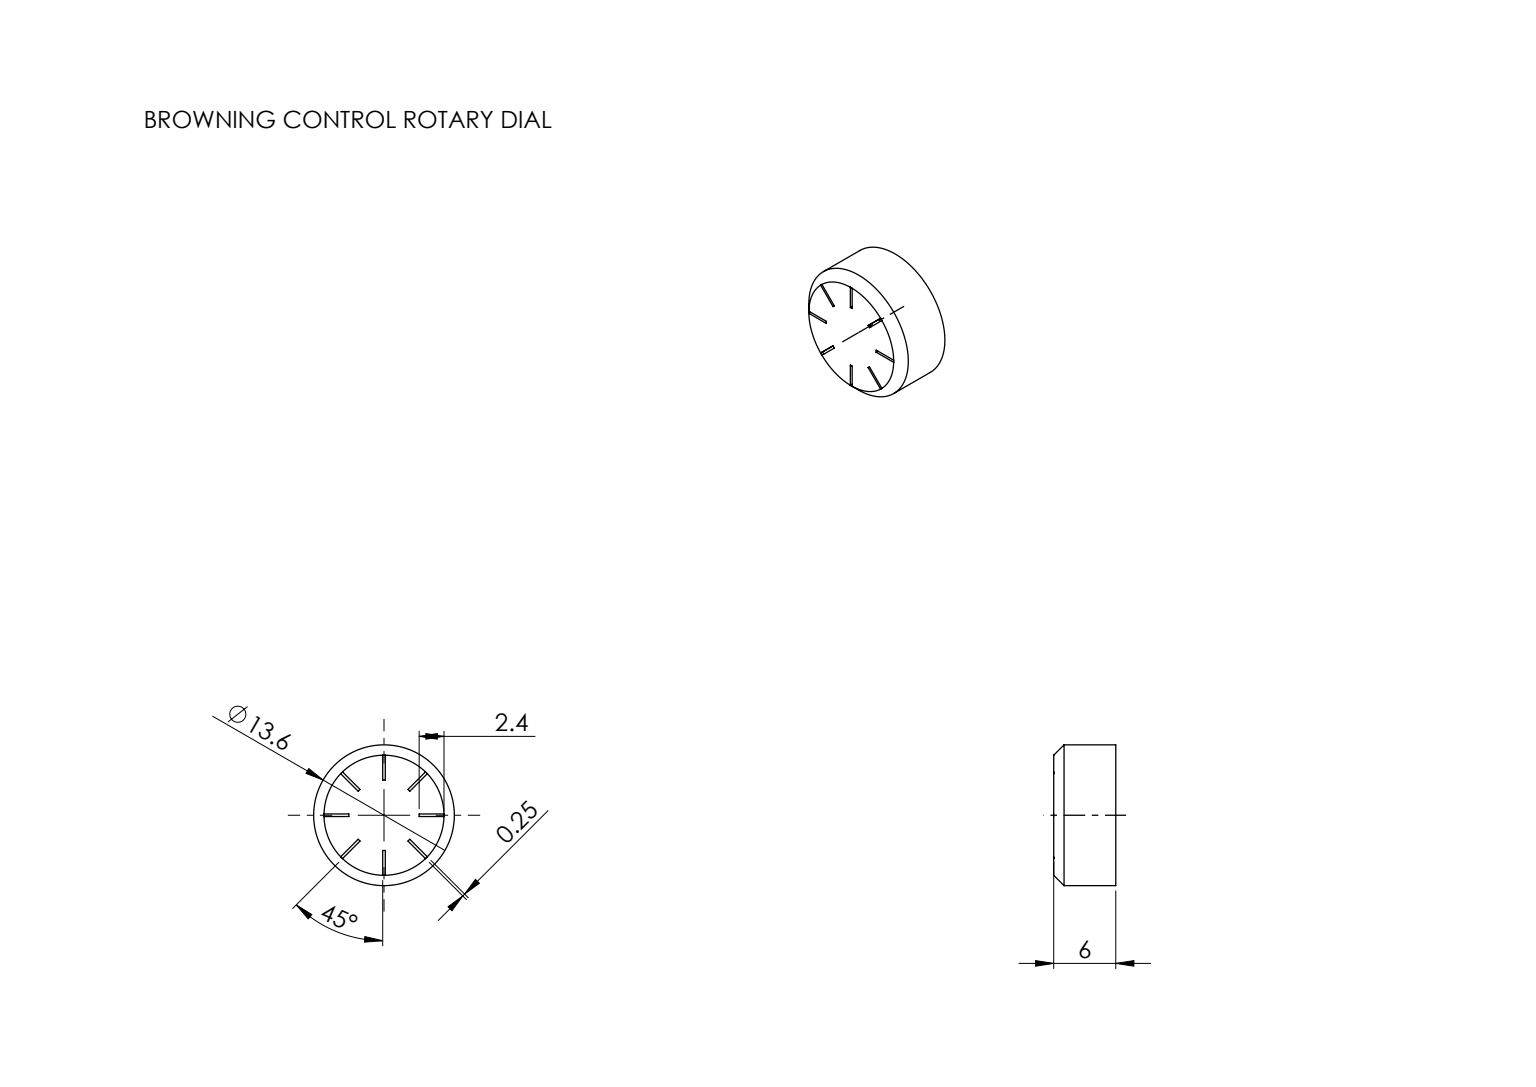
ISO-10303-21;
HEADER;
FILE_DESCRIPTION (('STEP AP214'),
    '1' );
FILE_NAME ('Browning Control Rotary Dial.step',
    '2026-10-08T14:41:38',
    ( '' ),
    ( '' ),
    'SwSTEP 2.0',
    'SolidWorks 2026',
    '' );
FILE_SCHEMA (( 'AUTOMOTIVE_DESIGN' ));
ENDSEC;

DATA;
#38=AXIS2_PLACEMENT_3D ( 'NONE', #15476, #386, #16855 ) ;
#44=EDGE_CURVE ( 'NONE', #885, #4327, #14471, .T. ) ;
#48=B_SPLINE_CURVE_WITH_KNOTS ( 'NONE', 3,
 ( #13537, #4634, #4733, #16687 ),
 .UNSPECIFIED., .F., .F.,
 ( 4, 4 ),
 ( 0.000000000000000000, 1.000000000000000000 ),
 .UNSPECIFIED. ) ;
#78=ADVANCED_FACE ( 'NONE', ( #3019 ), #8997, .T. ) ;
#88=CLOSED_SHELL ( 'NONE', ( #433, #16433, #12643, #3854, #16960, #8083, #12476, #2887, #13363, #11571, #11070, #10821, #5435, #14081, #18479, #16340, #3288, #10464, #13954, #1717, #18414, #1458, #6350, #11815, #16187, #14084, #2136, #6137, #1464, #12159, #2663, #1129, #18269, #562, #5420, #78, #10177, #12810, #725, #8545, #7974, #4556, #12238, #18488, #11655, #2010 ) ) ;
#89=VERTEX_POINT ( 'NONE', #13508 ) ;
#93=CARTESIAN_POINT ( 'NONE',  ( 4.072081901468762588, 26.82127119883315558, 59.66337542264481186 ) ) ;
#97=ORIENTED_EDGE ( 'NONE', *, *, #1658, .T. ) ;
#106=VERTEX_POINT ( 'NONE', #9669 ) ;
#125=CARTESIAN_POINT ( 'NONE',  ( 4.101219330881969327, 32.64264068711926825, 53.84264068711931372 ) ) ;
#154=PLANE ( 'NONE',  #4763 ) ;
#166=DIRECTION ( 'NONE',  ( 0.000000000000000000, -0.7071067811865495711, 0.7071067811865454633 ) ) ;
#181=ORIENTED_EDGE ( 'NONE', *, *, #18284, .T. ) ;
#182=ORIENTED_EDGE ( 'NONE', *, *, #1003, .F. ) ;
#191=CARTESIAN_POINT ( 'NONE',  ( 4.012354697599916697, 26.78000129688588871, 59.70432772728319293 ) ) ;
#212=ORIENTED_EDGE ( 'NONE', *, *, #12916, .T. ) ;
#217=EDGE_CURVE ( 'NONE', #3132, #14286, #15567, .T. ) ;
#224=ORIENTED_EDGE ( 'NONE', *, *, #676, .F. ) ;
#231=PLANE ( 'NONE',  #3745 ) ;
#237=DIRECTION ( 'NONE',  ( -0.7071067811865512365, -0.4999999999999988898, 0.4999999999999959477 ) ) ;
#239=DIRECTION ( 'NONE',  ( 0.7071067811865513475, 0.4999999999999988898, -0.4999999999999959477 ) ) ;
#256=DIRECTION ( 'NONE',  ( 0.000000000000000000, 0.7071067811865490160, -0.7071067811865461294 ) ) ;
#267=LINE ( 'NONE', #6253, #11429 ) ;
#275=DIRECTION ( 'NONE',  ( 0.000000000000000000, 0.7071067811865456854, 0.7071067811865494601 ) ) ;
#286=ORIENTED_EDGE ( 'NONE', *, *, #17624, .F. ) ;
#290=EDGE_LOOP ( 'NONE', ( #1568, #17362, #14195, #8849 ) ) ;
#305=ORIENTED_EDGE ( 'NONE', *, *, #2220, .F. ) ;
#314=EDGE_CURVE ( 'NONE', #106, #11781, #3884, .T. ) ;
#327=EDGE_CURVE ( 'NONE', #16495, #6094, #13076, .T. ) ;
#336=CARTESIAN_POINT ( 'NONE',  ( -1.084502282093227498E-14, 29.65425233947093986, 56.83102903476761725 ) ) ;
#357=CARTESIAN_POINT ( 'NONE',  ( -4.189607678530257395, 32.40336399182267257, 53.72836399182263278 ) ) ;
#386=DIRECTION ( 'NONE',  ( 0.000000000000000000, 0.7071067811865456854, 0.7071067811865494601 ) ) ;
#389=EDGE_LOOP ( 'NONE', ( #6259, #18026, #496, #1957 ) ) ;
#398=AXIS2_PLACEMENT_3D ( 'NONE', #14982, #7531, #3118 ) ;
#415=ORIENTED_EDGE ( 'NONE', *, *, #7089, .T. ) ;
#433=ADVANCED_FACE ( 'NONE', ( #10043 ), #844, .T. ) ;
#468=ORIENTED_EDGE ( 'NONE', *, *, #1195, .F. ) ;
#475=DIRECTION ( 'NONE',  ( -0.7071067811865511255, -0.4999999999999987788, 0.4999999999999958922 ) ) ;
#496=ORIENTED_EDGE ( 'NONE', *, *, #14059, .F. ) ;
#515=AXIS2_PLACEMENT_3D ( 'NONE', #7618, #13582, #166 ) ;
#521=CARTESIAN_POINT ( 'NONE',  ( 0.1249999999999895917, 33.84386001800125143, 52.64142135623733765 ) ) ;
#527=DIRECTION ( 'NONE',  ( -1.942890293094023946E-16, 0.7071067811865453523, 0.7071067811865496822 ) ) ;
#533=CARTESIAN_POINT ( 'NONE',  ( 4.101219330881941794, 26.84264068711924267, 59.64264068711931088 ) ) ;
#545=EDGE_CURVE ( 'NONE', #16762, #576, #17802, .T. ) ;
#562=ADVANCED_FACE ( 'NONE', ( #8873 ), #154, .T. ) ;
#563=ORIENTED_EDGE ( 'NONE', *, *, #6960, .T. ) ;
#576=VERTEX_POINT ( 'NONE', #13377 ) ;
#582=DIRECTION ( 'NONE',  ( 2.220446049250312834E-16, 0.7071067811865455743, 0.7071067811865493491 ) ) ;
#591=CARTESIAN_POINT ( 'NONE',  ( 5.799999999999985612, 29.65425233947092920, 56.47747564417436195 ) ) ;
#598=CARTESIAN_POINT ( 'NONE',  ( 5.799999999999985612, 29.65425233947092920, 56.47747564417436195 ) ) ;
#602=ORIENTED_EDGE ( 'NONE', *, *, #4334, .F. ) ;
#609=AXIS2_PLACEMENT_3D ( 'NONE', #15894, #14234, #2648 ) ;
#666=CARTESIAN_POINT ( 'NONE',  ( 5.799999999999985612, 29.65425233947092920, 56.47747564417436195 ) ) ;
#671=COLOUR_RGB ( '', 0.72549020, 0.75294118, 0.79215686) ;
#676=EDGE_CURVE ( 'NONE', #9708, #9275, #13573, .T. ) ;
#693=CARTESIAN_POINT ( 'NONE',  ( -1.040834085586084257E-14, 29.03553390593270578, 56.03553390593273775 ) ) ;
#704=CARTESIAN_POINT ( 'NONE',  ( -4.012354697599906928, 32.70432772728319293, 53.78000129688592068 ) ) ;
#705=CARTESIAN_POINT ( 'NONE',  ( -0.1250000000000104083, 31.97002704785689531, 54.16170093578840294 ) ) ;
#706=EDGE_CURVE ( 'NONE', #9890, #18408, #2462, .T. ) ;
#716=CARTESIAN_POINT ( 'NONE',  ( -2.492551403682565780, 31.20336399182265552, 54.92836399182263563 ) ) ;
#725=ADVANCED_FACE ( 'NONE', ( #16824 ), #4868, .T. ) ;
#742=DIRECTION ( 'NONE',  ( -1.000000000000000000, 2.720046410331633524E-15, -2.220446049250313081E-15 ) ) ;
#750=ORIENTED_EDGE ( 'NONE', *, *, #15854, .T. ) ;
#779=ORIENTED_EDGE ( 'NONE', *, *, #9790, .T. ) ;
#789=FACE_OUTER_BOUND ( 'NONE', #10775, .T. ) ;
#807=FACE_OUTER_BOUND ( 'NONE', #12482, .T. ) ;
#816=ORIENTED_EDGE ( 'NONE', *, *, #9598, .T. ) ;
#835=SURFACE_STYLE_FILL_AREA ( #11035 ) ;
#842=ORIENTED_EDGE ( 'NONE', *, *, #15989, .T. ) ;
#843=FACE_OUTER_BOUND ( 'NONE', #12229, .T. ) ;
#844=CYLINDRICAL_SURFACE ( 'NONE', #14759, 6.799999999999997158 ) ;
#852=LINE ( 'NONE', #17325, #17405 ) ;
#861=EDGE_CURVE ( 'NONE', #12841, #2217, #5438, .T. ) ;
#872=DIRECTION ( 'NONE',  ( 0.5773502691896360561, 0.8164965809277188180, 0.000000000000000000 ) ) ;
#881=ORIENTED_EDGE ( 'NONE', *, *, #9499, .T. ) ;
#885=VERTEX_POINT ( 'NONE', #10021 ) ;
#889=CARTESIAN_POINT ( 'NONE',  ( 0.1249999999999895917, 27.16170093578836031, 58.97002704785691662 ) ) ;
#895=VERTEX_POINT ( 'NONE', #3865 ) ;
#903=DIRECTION ( 'NONE',  ( 1.000000000000000000, -7.410738689372937262E-15, 7.410738689372897819E-15 ) ) ;
#914=DIRECTION ( 'NONE',  ( 1.000000000000000000, -2.665111688417744333E-15, 2.272588573746785565E-15 ) ) ;
#989=CARTESIAN_POINT ( 'NONE',  ( -5.799326430397251819, 29.65377616443625541, 56.83055285973284754 ) ) ;
#990=ORIENTED_EDGE ( 'NONE', *, *, #7649, .F. ) ;
#1003=EDGE_CURVE ( 'NONE', #16765, #16368, #9344, .T. ) ;
#1051=ORIENTED_EDGE ( 'NONE', *, *, #5788, .F. ) ;
#1061=DIRECTION ( 'NONE',  ( -0.000000000000000000, 0.7071067811865493491, -0.7071067811865456854 ) ) ;
#1068=CARTESIAN_POINT ( 'NONE',  ( -9.575581032440643243E-15, 20.69167388793145079, 57.30832611206850657 ) ) ;
#1072=ORIENTED_EDGE ( 'NONE', *, *, #15999, .T. ) ;
#1092=EDGE_CURVE ( 'NONE', #2343, #576, #12483, .T. ) ;
#1097=ORIENTED_EDGE ( 'NONE', *, *, #3003, .F. ) ;
#1128=AXIS2_PLACEMENT_3D ( 'NONE', #9817, #18860, #10100 ) ;
#1129=ADVANCED_FACE ( 'NONE', ( #7187 ), #13161, .F. ) ;
#1140=CARTESIAN_POINT ( 'NONE',  ( 4.189607678530260948, 26.72836399182260791, 59.40336399182267257 ) ) ;
#1157=CARTESIAN_POINT ( 'NONE',  ( -4.160453206537193083, 26.88344170207934525, 59.60057016663802187 ) ) ;
#1163=CARTESIAN_POINT ( 'NONE',  ( -5.800000000000006928, 29.47747564417435484, 56.65425233947093631 ) ) ;
#1169=ORIENTED_EDGE ( 'NONE', *, *, #14932, .T. ) ;
#1170=ORIENTED_EDGE ( 'NONE', *, *, #17994, .F. ) ;
#1175=DIRECTION ( 'NONE',  ( 0.7071067811865388020, -0.5000000000000074385, 0.5000000000000046629 ) ) ;
#1176=ORIENTED_EDGE ( 'NONE', *, *, #1238, .T. ) ;
#1185=SHAPE_DEFINITION_REPRESENTATION ( #6159, #2502 ) ;
#1189=LINE ( 'NONE', #8840, #18689 ) ;
#1191=ORIENTED_EDGE ( 'NONE', *, *, #676, .T. ) ;
#1195=EDGE_CURVE ( 'NONE', #4388, #12056, #11985, .T. ) ;
#1201=DIRECTION ( 'NONE',  ( -2.775557561562890858E-16, 0.7071067811865456854, 0.7071067811865493491 ) ) ;
#1221=DIRECTION ( 'NONE',  ( -0.5773502691896282846, -0.8164965809277242581, 0.000000000000000000 ) ) ;
#1231=CARTESIAN_POINT ( 'NONE',  ( 0.1249999999999895917, 25.46464466094064250, 60.66708332270462734 ) ) ;
#1232=DIRECTION ( 'NONE',  ( 0.7071067811865414665, -0.5000000000000058842, 0.5000000000000028866 ) ) ;
#1235=LINE ( 'NONE', #1140, #3481 ) ;
#1238=EDGE_CURVE ( 'NONE', #3008, #10469, #14216, .T. ) ;
#1256=EDGE_LOOP ( 'NONE', ( #16470, #14104, #2812, #8914 ) ) ;
#1263=DIRECTION ( 'NONE',  ( 0.000000000000000000, -0.7071067811865452413, -0.7071067811865497932 ) ) ;
#1268=CARTESIAN_POINT ( 'NONE',  ( -0.1250000000000104083, 27.33847763108499507, 59.14680374315354783 ) ) ;
#1292=CARTESIAN_POINT ( 'NONE',  ( -2.492551403682614186, 28.10514068711927749, 58.38014068711927251 ) ) ;
#1297=CARTESIAN_POINT ( 'NONE',  ( -2.315774708385926139, 31.50514068711928672, 54.98014068711927393 ) ) ;
#1325=VECTOR ( 'NONE', #4373, 1000.000000000000114 ) ;
#1339=B_SPLINE_CURVE_WITH_KNOTS ( 'NONE', 3,
 ( #8067, #10986, #6398, #704 ),
 .UNSPECIFIED., .F., .F.,
 ( 4, 4 ),
 ( 0.000000000000000000, 1.000000000000000000 ),
 .UNSPECIFIED. ) ;
#1340=DIRECTION ( 'NONE',  ( 0.000000000000000000, -0.7071067811865457964, -0.7071067811865492381 ) ) ;
#1349=ORIENTED_EDGE ( 'NONE', *, *, #2635, .F. ) ;
#1357=ORIENTED_EDGE ( 'NONE', *, *, #4764, .F. ) ;
#1360=EDGE_CURVE ( 'NONE', #16495, #18191, #17257, .T. ) ;
#1375=EDGE_LOOP ( 'NONE', ( #3971, #16864, #9192, #16577, #12901 ) ) ;
#1378=CARTESIAN_POINT ( 'NONE',  ( -4.012354697599992193, 26.78000129688593134, 59.70432772728315740 ) ) ;
#1388=CARTESIAN_POINT ( 'NONE',  ( -4.189607678530257395, 32.40336399182267257, 53.72836399182263278 ) ) ;
#1432=DIRECTION ( 'NONE',  ( 1.000000000000000000, 0.000000000000000000, -0.000000000000000000 ) ) ;
#1447=VERTEX_POINT ( 'NONE', #12922 ) ;
#1458=ADVANCED_FACE ( 'NONE', ( #15877 ), #16253, .F. ) ;
#1463=CARTESIAN_POINT ( 'NONE',  ( 4.101219330881969327, 32.64264068711926825, 53.84264068711931372 ) ) ;
#1464=ADVANCED_FACE ( 'NONE', ( #18916 ), #11445, .T. ) ;
#1486=ORIENTED_EDGE ( 'NONE', *, *, #7089, .F. ) ;
#1491=CARTESIAN_POINT ( 'NONE',  ( -0.1250000000000104083, 25.46464466094064250, 60.66708332270462734 ) ) ;
#1539=LINE ( 'NONE', #7513, #3636 ) ;
#1555=LINE ( 'NONE', #17724, #16314 ) ;
#1559=CARTESIAN_POINT ( 'NONE',  ( 2.315774708385922587, 27.80336399182260720, 58.32836399182267684 ) ) ;
#1562=CARTESIAN_POINT ( 'NONE',  ( 4.042620306204053549, 26.80012125920691446, 59.68389060951044200 ) ) ;
#1564=EDGE_CURVE ( 'NONE', #16934, #16046, #11536, .T. ) ;
#1568=ORIENTED_EDGE ( 'NONE', *, *, #12470, .F. ) ;
#1607=VERTEX_POINT ( 'NONE', #1463 ) ;
#1640=AXIS2_PLACEMENT_3D ( 'NONE', #2314, #2693, #1221 ) ;
#1658=EDGE_CURVE ( 'NONE', #6570, #18891, #1755, .T. ) ;
#1664=FACE_OUTER_BOUND ( 'NONE', #7252, .T. ) ;
#1669=ORIENTED_EDGE ( 'NONE', *, *, #17624, .T. ) ;
#1688=CARTESIAN_POINT ( 'NONE',  ( -0.1250000000000104083, 25.46464466094064250, 60.66708332270462734 ) ) ;
#1692=EDGE_LOOP ( 'NONE', ( #8443, #17446, #17916, #6022 ) ) ;
#1694=CARTESIAN_POINT ( 'NONE',  ( 0.000000000000000000, 43.06586399182256741, 43.06586399182279479 ) ) ;
#1700=LINE ( 'NONE', #15233, #14879 ) ;
#1702=EDGE_CURVE ( 'NONE', #16934, #9890, #16362, .T. ) ;
#1708=FACE_OUTER_BOUND ( 'NONE', #5051, .T. ) ;
#1714=EDGE_CURVE ( 'NONE', #13315, #14325, #16755, .T. ) ;
#1717=ADVANCED_FACE ( 'NONE', ( #1664 ), #14985, .T. ) ;
#1724=DIRECTION ( 'NONE',  ( 0.7071067811865513475, 0.4999999999999988898, -0.4999999999999959477 ) ) ;
#1755=LINE ( 'NONE', #19303, #8738 ) ;
#1789=VERTEX_POINT ( 'NONE', #4898 ) ;
#1791=AXIS2_PLACEMENT_3D ( 'NONE', #13713, #4815, #7646 ) ;
#1801=LINE ( 'NONE', #3561, #9692 ) ;
#1809=VERTEX_POINT ( 'NONE', #18426 ) ;
#1810=B_SPLINE_CURVE_WITH_KNOTS ( 'NONE', 3,
 ( #6841, #15227, #8048, #2057 ),
 .UNSPECIFIED., .F., .F.,
 ( 4, 4 ),
 ( 0.000000000000000000, 1.000000000000000000 ),
 .UNSPECIFIED. ) ;
#1812=EDGE_CURVE ( 'NONE', #17726, #12801, #3518, .T. ) ;
#1823=DIRECTION ( 'NONE',  ( -0.5773502691896228445, 0.8164965809277280329, 0.000000000000000000 ) ) ;
#1830=DIRECTION ( 'NONE',  ( -0.7071067811865437980, 0.5000000000000039968, -0.5000000000000013323 ) ) ;
#1901=DIRECTION ( 'NONE',  ( -0.7071067811865537900, -0.4999999999999972800, 0.4999999999999940603 ) ) ;
#1957=ORIENTED_EDGE ( 'NONE', *, *, #3607, .F. ) ;
#1965=AXIS2_PLACEMENT_3D ( 'NONE', #17931, #275, #5869 ) ;
#1973=FACE_OUTER_BOUND ( 'NONE', #5364, .T. ) ;
#2010=ADVANCED_FACE ( 'NONE', ( #14469 ), #14659, .T. ) ;
#2035=ORIENTED_EDGE ( 'NONE', *, *, #2635, .T. ) ;
#2043=CARTESIAN_POINT ( 'NONE',  ( -2.315774708385978098, 27.80336399182263563, 58.32836399182264131 ) ) ;
#2051=VECTOR ( 'NONE', #14820, 1000.000000000000000 ) ;
#2057=CARTESIAN_POINT ( 'NONE',  ( 5.799326430397229615, 29.65377616443619857, 56.83055285973290438 ) ) ;
#2067=LINE ( 'NONE', #7958, #15703 ) ;
#2078=DIRECTION ( 'NONE',  ( -7.602811950582247805E-15, 0.000000000000000000, 1.000000000000000000 ) ) ;
#2080=VERTEX_POINT ( 'NONE', #12985 ) ;
#2093=ORIENTED_EDGE ( 'NONE', *, *, #11143, .F. ) ;
#2094=DIRECTION ( 'NONE',  ( 8.659560562354847809E-17, -1.000000000000000000, -1.221245327087672194E-14 ) ) ;
#2097=DIRECTION ( 'NONE',  ( 0.000000000000000000, 0.7071067811865456854, 0.7071067811865494601 ) ) ;
#2119=CARTESIAN_POINT ( 'NONE',  ( -3.400000000000017675, 29.47747564417433352, 56.65425233947095052 ) ) ;
#2136=ADVANCED_FACE ( 'NONE', ( #8678 ), #2411, .F. ) ;
#2188=CARTESIAN_POINT ( 'NONE',  ( 4.012830983233651061, 32.52836399182262994, 53.60336399182268252 ) ) ;
#2191=CARTESIAN_POINT ( 'NONE',  ( -13.49999999999974065, 39.11180553784110003, 47.01992244580424085 ) ) ;
#2195=CIRCLE ( 'NONE', #4064, 6.799999999999999822 ) ;
#2201=FACE_OUTER_BOUND ( 'NONE', #18242, .T. ) ;
#2217=VERTEX_POINT ( 'NONE', #6047 ) ;
#2220=EDGE_CURVE ( 'NONE', #10469, #11653, #13483, .T. ) ;
#2236=DIRECTION ( 'NONE',  ( -2.220446049250312588E-16, 0.7071067811865453523, 0.7071067811865496822 ) ) ;
#2243=ORIENTED_EDGE ( 'NONE', *, *, #4334, .T. ) ;
#2261=CARTESIAN_POINT ( 'NONE',  ( -4.189131392896543460, 32.57932772728320003, 53.90500129688591358 ) ) ;
#2279=ORIENTED_EDGE ( 'NONE', *, *, #9499, .F. ) ;
#2281=VERTEX_POINT ( 'NONE', #13274 ) ;
#2288=CARTESIAN_POINT ( 'NONE',  ( 2.492551403682577771, 31.20336399182262710, 54.92836399182266405 ) ) ;
#2295=CARTESIAN_POINT ( 'NONE',  ( -0.1250000000000104083, 27.33847763108499507, 59.14680374315354783 ) ) ;
#2304=CARTESIAN_POINT ( 'NONE',  ( 5.800448907431066559, 29.80092238452519382, 56.68308948419219462 ) ) ;
#2314=CARTESIAN_POINT ( 'NONE',  ( 4.012830983233651061, 32.52836399182262994, 53.60336399182268252 ) ) ;
#2343=VERTEX_POINT ( 'NONE', #8203 ) ;
#2355=PRODUCT_DEFINITION_FORMATION_WITH_SPECIFIED_SOURCE ( 'ANY', '', #17717, .NOT_KNOWN. ) ;
#2371=DIRECTION ( 'NONE',  ( 0.5773502691896202910, -0.8164965809277299202, 0.000000000000000000 ) ) ;
#2373=CARTESIAN_POINT ( 'NONE',  ( -2.492551403682614186, 27.92836399182264273, 58.20336399182264131 ) ) ;
#2382=EDGE_LOOP ( 'NONE', ( #2833, #842, #12674, #5103 ) ) ;
#2386=CARTESIAN_POINT ( 'NONE',  ( -3.400000000000017675, 29.65425233947097183, 56.47747564417432642 ) ) ;
#2399=LINE ( 'NONE', #17121, #17102 ) ;
#2400=ORIENTED_EDGE ( 'NONE', *, *, #2495, .T. ) ;
#2411=PLANE ( 'NONE',  #15954 ) ;
#2417=ORIENTED_EDGE ( 'NONE', *, *, #8519, .T. ) ;
#2432=EDGE_CURVE ( 'NONE', #4388, #16762, #11119, .T. ) ;
#2447=VECTOR ( 'NONE', #6633, 999.9999999999998863 ) ;
#2462=CIRCLE ( 'NONE', #15927, 5.800000000000007816 ) ;
#2485=CARTESIAN_POINT ( 'NONE',  ( -5.800448837981397432, 29.77177811653248796, 56.71286850494549014 ) ) ;
#2495=EDGE_CURVE ( 'NONE', #2080, #15466, #3013, .T. ) ;
#2502=SHAPE_REPRESENTATION ( 'Browning Control Rotary Dial', ( #1791 ), #2636 ) ;
#2503=DIRECTION ( 'NONE',  ( 0.000000000000000000, 0.7071067811865456854, 0.7071067811865494601 ) ) ;
#2521=ORIENTED_EDGE ( 'NONE', *, *, #16911, .F. ) ;
#2544=ORIENTED_EDGE ( 'NONE', *, *, #706, .F. ) ;
#2549=EDGE_CURVE ( 'NONE', #5878, #3990, #9749, .T. ) ;
#2556=ORIENTED_EDGE ( 'NONE', *, *, #4085, .T. ) ;
#2562=VECTOR ( 'NONE', #7706, 1000.000000000000000 ) ;
#2578=CARTESIAN_POINT ( 'NONE',  ( -2.315774708385926139, 31.32836399182264842, 54.80336399182263563 ) ) ;
#2607=ORIENTED_EDGE ( 'NONE', *, *, #14511, .T. ) ;
#2635=EDGE_CURVE ( 'NONE', #9275, #12801, #2195, .T. ) ;
#2636=( GEOMETRIC_REPRESENTATION_CONTEXT ( 3 ) GLOBAL_UNCERTAINTY_ASSIGNED_CONTEXT ( ( #16291 ) ) GLOBAL_UNIT_ASSIGNED_CONTEXT ( ( #11213, #5357, #8294 ) ) REPRESENTATION_CONTEXT ( 'NONE', 'WORKASPACE' ) );
#2648=DIRECTION ( 'NONE',  ( -2.665111688417744333E-15, -1.000000000000000000, 0.000000000000000000 ) ) ;
#2654=AXIS2_PLACEMENT_3D ( 'NONE', #5320, #4141, #13134 ) ;
#2657=EDGE_CURVE ( 'NONE', #895, #7943, #12290, .T. ) ;
#2662=ORIENTED_EDGE ( 'NONE', *, *, #15902, .T. ) ;
#2663=ADVANCED_FACE ( 'NONE', ( #6513 ), #18184, .T. ) ;
#2672=CARTESIAN_POINT ( 'NONE',  ( 4.160453206537142457, 32.60057016663802187, 53.88344170207938788 ) ) ;
#2690=VERTEX_POINT ( 'NONE', #7653 ) ;
#2693=DIRECTION ( 'NONE',  ( -0.7071067811865463515, 0.5000000000000024425, -0.4999999999999993339 ) ) ;
#2696=CONICAL_SURFACE ( 'NONE', #13654, 5.800000000000005151, 0.7853981633974385090 ) ;
#2701=DIRECTION ( 'NONE',  ( -0.000000000000000000, -0.7071067811865456854, -0.7071067811865494601 ) ) ;
#2711=ORIENTED_EDGE ( 'NONE', *, *, #9387, .F. ) ;
#2730=CARTESIAN_POINT ( 'NONE',  ( -0.1250000000000104083, 27.16170093578836031, 58.97002704785691662 ) ) ;
#2767=DIRECTION ( 'NONE',  ( 0.7071067811865512365, 0.4999999999999988898, -0.4999999999999959477 ) ) ;
#2769=DIRECTION ( 'NONE',  ( 0.000000000000000000, -0.7071067811865454633, -0.7071067811865496822 ) ) ;
#2772=PLANE ( 'NONE',  #13601 ) ;
#2774=CARTESIAN_POINT ( 'NONE',  ( 0.1249999999999895917, 25.46464466094064250, 60.66708332270462734 ) ) ;
#2781=CARTESIAN_POINT ( 'NONE',  ( -5.799326430397249155, 29.83055285973289372, 56.65377616443620212 ) ) ;
#2811=CARTESIAN_POINT ( 'NONE',  ( -9.971658890789427512E-15, 29.83102903476757817, 56.65425233947097894 ) ) ;
#2812=ORIENTED_EDGE ( 'NONE', *, *, #3312, .T. ) ;
#2819=ORIENTED_EDGE ( 'NONE', *, *, #8356, .F. ) ;
#2822=ORIENTED_EDGE ( 'NONE', *, *, #14511, .F. ) ;
#2823=ORIENTED_EDGE ( 'NONE', *, *, #14262, .F. ) ;
#2825=DIRECTION ( 'NONE',  ( 0.000000000000000000, -0.7071067811865497932, 0.7071067811865452413 ) ) ;
#2826=DIRECTION ( 'NONE',  ( 0.000000000000000000, -0.7071067811865454633, -0.7071067811865496822 ) ) ;
#2833=ORIENTED_EDGE ( 'NONE', *, *, #14108, .F. ) ;
#2883=DIRECTION ( 'NONE',  ( -2.775557561562890858E-16, 0.7071067811865454633, 0.7071067811865496822 ) ) ;
#2887=ADVANCED_FACE ( 'NONE', ( #10384 ), #11750, .T. ) ;
#2895=CARTESIAN_POINT ( 'NONE',  ( 0.1249999999999895917, 33.84290755733280065, 52.64142146683631296 ) ) ;
#2928=EDGE_CURVE ( 'NONE', #12056, #2690, #12635, .T. ) ;
#2929=CARTESIAN_POINT ( 'NONE',  ( 0.08838834764830766355, 29.80514068711926257, 56.68014068711929809 ) ) ;
#2930=CARTESIAN_POINT ( 'NONE',  ( -1.040834085586084257E-14, 33.84386001800124433, 51.22720779386423118 ) ) ;
#2950=PLANE ( 'NONE',  #16446 ) ;
#3003=EDGE_CURVE ( 'NONE', #17432, #18408, #4914, .T. ) ;
#3008=VERTEX_POINT ( 'NONE', #18544 ) ;
#3013=B_SPLINE_CURVE_WITH_KNOTS ( 'NONE', 3,
 ( #11207, #2485, #17481, #8287 ),
 .UNSPECIFIED., .F., .F.,
 ( 4, 4 ),
 ( 0.000000000000000000, 1.000000000000000000 ),
 .UNSPECIFIED. ) ;
#3016=ORIENTED_EDGE ( 'NONE', *, *, #9343, .F. ) ;
#3019=FACE_OUTER_BOUND ( 'NONE', #17852, .T. ) ;
#3063=CARTESIAN_POINT ( 'NONE',  ( 0.04165538583019261221, 25.64078660347668759, 60.84386001800125854 ) ) ;
#3086=CARTESIAN_POINT ( 'NONE',  ( -2.315774708385926139, 31.50514068711928672, 54.98014068711927393 ) ) ;
#3091=CARTESIAN_POINT ( 'NONE',  ( 0.1249999999999895917, 32.14680374315353362, 54.33847763108504125 ) ) ;
#3118=DIRECTION ( 'NONE',  ( -1.000000000000000000, 0.000000000000000000, 0.000000000000000000 ) ) ;
#3129=ORIENTED_EDGE ( 'NONE', *, *, #15264, .F. ) ;
#3131=CARTESIAN_POINT ( 'NONE',  ( -0.1250000000000104083, 33.66708332270461312, 52.46464466094069934 ) ) ;
#3132=VERTEX_POINT ( 'NONE', #18721 ) ;
#3160=STYLED_ITEM ( 'NONE', ( #4954 ), #10129 ) ;
#3165=CARTESIAN_POINT ( 'NONE',  ( 4.072081901468789233, 32.66337542264476923, 53.82127119883322308 ) ) ;
#3177=VECTOR ( 'NONE', #18325, 1000.000000000000114 ) ;
#3212=ORIENTED_EDGE ( 'NONE', *, *, #1238, .F. ) ;
#3220=ORIENTED_EDGE ( 'NONE', *, *, #15244, .T. ) ;
#3265=CARTESIAN_POINT ( 'NONE',  ( 2.315774708385941683, 31.32836399182263065, 54.80336399182266405 ) ) ;
#3270=LINE ( 'NONE', #521, #14377 ) ;
#3277=CARTESIAN_POINT ( 'NONE',  ( -13.50000000000003908, 20.01992244580436164, 66.11180553784085134 ) ) ;
#3280=( LENGTH_UNIT ( ) NAMED_UNIT ( * ) SI_UNIT ( .MILLI., .METRE. ) );
#3288=ADVANCED_FACE ( 'NONE', ( #18518 ), #8557, .F. ) ;
#3309=ORIENTED_EDGE ( 'NONE', *, *, #6175, .T. ) ;
#3312=EDGE_CURVE ( 'NONE', #13315, #11055, #8650, .T. ) ;
#3343=ORIENTED_EDGE ( 'NONE', *, *, #327, .T. ) ;
#3370=DIRECTION ( 'NONE',  ( -1.047444401652940007E-14, -0.7071067811865495711, 0.7071067811865454633 ) ) ;
#3422=EDGE_LOOP ( 'NONE', ( #2521, #2243, #13517, #11831 ) ) ;
#3427=ORIENTED_EDGE ( 'NONE', *, *, #16911, .T. ) ;
#3444=VECTOR ( 'NONE', #1201, 1000.000000000000114 ) ;
#3448=FACE_OUTER_BOUND ( 'NONE', #7421, .T. ) ;
#3459=AXIS2_PLACEMENT_3D ( 'NONE', #693, #6677, #16627 ) ;
#3462=ORIENTED_EDGE ( 'NONE', *, *, #12015, .F. ) ;
#3481=VECTOR ( 'NONE', #17234, 1000.000000000000000 ) ;
#3514=VECTOR ( 'NONE', #582, 1000.000000000000114 ) ;
#3517=FACE_OUTER_BOUND ( 'NONE', #7642, .T. ) ;
#3518=LINE ( 'NONE', #12706, #18159 ) ;
#3558=EDGE_LOOP ( 'NONE', ( #10549, #14712, #6356, #14505, #17843, #2544, #4769, #3309, #10055, #12014, #9614, #182, #6932, #5407, #8428 ) ) ;
#3561=CARTESIAN_POINT ( 'NONE',  ( -0.1250000000000104083, 27.16170093578836031, 58.97002704785691662 ) ) ;
#3564=CARTESIAN_POINT ( 'NONE',  ( -1.040834085586084257E-14, 25.49999999999998934, 52.50000000000000000 ) ) ;
#3607=EDGE_CURVE ( 'NONE', #19340, #17432, #18467, .T. ) ;
#3631=DIRECTION ( 'NONE',  ( 0.000000000000000000, 0.7071067811865490160, -0.7071067811865461294 ) ) ;
#3635=CARTESIAN_POINT ( 'NONE',  ( 3.399999999999996803, 29.47747564417430155, 56.65425233947098604 ) ) ;
#3636=VECTOR ( 'NONE', #12113, 1000.000000000000227 ) ;
#3655=ORIENTED_EDGE ( 'NONE', *, *, #5788, .T. ) ;
#3699=DIRECTION ( 'NONE',  ( -0.000000000000000000, -0.7071067811865456854, -0.7071067811865493491 ) ) ;
#3708=ORIENTED_EDGE ( 'NONE', *, *, #13973, .F. ) ;
#3714=PLANE ( 'NONE',  #9451 ) ;
#3745=AXIS2_PLACEMENT_3D ( 'NONE', #4252, #17774, #2769 ) ;
#3760=AXIS2_PLACEMENT_3D ( 'NONE', #16578, #16482, #10485 ) ;
#3765=VECTOR ( 'NONE', #15296, 1000.000000000000114 ) ;
#3786=ORIENTED_EDGE ( 'NONE', *, *, #6175, .F. ) ;
#3798=DIRECTION ( 'NONE',  ( 2.775557561562890858E-16, 0.7071067811865454633, 0.7071067811865496822 ) ) ;
#3825=DIRECTION ( 'NONE',  ( 3.491481338843133355E-15, 0.7071067811865495711, -0.7071067811865454633 ) ) ;
#3839=DIRECTION ( 'NONE',  ( 0.000000000000000000, -0.7071067811865495711, 0.7071067811865454633 ) ) ;
#3844=ORIENTED_EDGE ( 'NONE', *, *, #13213, .T. ) ;
#3854=ADVANCED_FACE ( 'NONE', ( #13423 ), #5995, .T. ) ;
#3855=DIRECTION ( 'NONE',  ( -0.5773502691896255090, 0.8164965809277261455, 0.000000000000000000 ) ) ;
#3865=CARTESIAN_POINT ( 'NONE',  ( 4.189607678530260948, 26.72836399182260791, 59.40336399182267257 ) ) ;
#3884=LINE ( 'NONE', #14467, #9743 ) ;
#3913=CARTESIAN_POINT ( 'NONE',  ( 4.012830983233625304, 26.60336399182260791, 59.52836399182266547 ) ) ;
#3914=DIRECTION ( 'NONE',  ( 0.5773502691896335026, 0.8164965809277204833, 0.000000000000000000 ) ) ;
#3964=AXIS2_PLACEMENT_3D ( 'NONE', #15505, #6775, #2078 ) ;
#3971=ORIENTED_EDGE ( 'NONE', *, *, #16201, .F. ) ;
#3980=ORIENTED_EDGE ( 'NONE', *, *, #11178, .T. ) ;
#3990=VERTEX_POINT ( 'NONE', #9505 ) ;
#4007=CARTESIAN_POINT ( 'NONE',  ( 0.1249999999999895917, 32.14680374315353362, 54.33847763108504125 ) ) ;
#4027=LINE ( 'NONE', #12754, #17835 ) ;
#4057=APPLICATION_CONTEXT ( 'automotive_design' ) ;
#4061=LINE ( 'NONE', #9751, #5852 ) ;
#4064=AXIS2_PLACEMENT_3D ( 'NONE', #3564, #2097, #7787 ) ;
#4065=ORIENTED_EDGE ( 'NONE', *, *, #17882, .T. ) ;
#4085=EDGE_CURVE ( 'NONE', #5200, #8744, #13461, .T. ) ;
#4088=ORIENTED_EDGE ( 'NONE', *, *, #17527, .F. ) ;
#4106=CARTESIAN_POINT ( 'NONE',  ( -4.130991513055715103, 32.62172003681460808, 53.86292658466337713 ) ) ;
#4127=ORIENTED_EDGE ( 'NONE', *, *, #15999, .F. ) ;
#4141=DIRECTION ( 'NONE',  ( -0.7071067811865562325, -0.4999999999999955036, 0.4999999999999924505 ) ) ;
#4150=ORIENTED_EDGE ( 'NONE', *, *, #7742, .F. ) ;
#4157=CARTESIAN_POINT ( 'NONE',  ( -4.189607678530257395, 32.40336399182267257, 53.72836399182263278 ) ) ;
#4194=ORIENTED_EDGE ( 'NONE', *, *, #13010, .F. ) ;
#4234=DIRECTION ( 'NONE',  ( 0.5773502691896311712, 0.8164965809277222597, 0.000000000000000000 ) ) ;
#4252=CARTESIAN_POINT ( 'NONE',  ( -5.800000000000006928, 29.65425233947099315, 56.47747564417430510 ) ) ;
#4301=CARTESIAN_POINT ( 'NONE',  ( -4.189131392896629613, 26.90500129688593134, 59.57932772728315030 ) ) ;
#4311=LINE ( 'NONE', #10467, #8937 ) ;
#4320=CARTESIAN_POINT ( 'NONE',  ( -0.08838834764833139457, 29.68014068711926257, 56.80514068711929809 ) ) ;
#4322=VERTEX_POINT ( 'NONE', #7236 ) ;
#4327=VERTEX_POINT ( 'NONE', #8895 ) ;
#4329=LINE ( 'NONE', #1292, #2051 ) ;
#4334=EDGE_CURVE ( 'NONE', #16046, #5763, #1555, .T. ) ;
#4353=EDGE_CURVE ( 'NONE', #17254, #2217, #12488, .T. ) ;
#4357=DIRECTION ( 'NONE',  ( 1.000000000000000000, 0.000000000000000000, -0.000000000000000000 ) ) ;
#4361=VECTOR ( 'NONE', #17532, 1000.000000000000000 ) ;
#4363=CARTESIAN_POINT ( 'NONE',  ( 4.101219330881941794, 26.84264068711924267, 59.64264068711931088 ) ) ;
#4365=ORIENTED_EDGE ( 'NONE', *, *, #2928, .T. ) ;
#4370=AXIS2_PLACEMENT_3D ( 'NONE', #14648, #17691, #10124 ) ;
#4373=DIRECTION ( 'NONE',  ( -0.7071067811865486830, -0.5000000000000005551, 0.4999999999999978351 ) ) ;
#4384=CARTESIAN_POINT ( 'NONE',  ( 5.799326430397229615, 29.65377616443619857, 56.83055285973290438 ) ) ;
#4388=VERTEX_POINT ( 'NONE', #11045 ) ;
#4390=CONICAL_SURFACE ( 'NONE', #16923, 5.800000000000005151, 0.7853981633974385090 ) ;
#4400=EDGE_LOOP ( 'NONE', ( #18506, #15112, #16402, #3016, #13450 ) ) ;
#4402=CARTESIAN_POINT ( 'NONE',  ( -4.130991513055792375, 26.86292658466339489, 59.62172003681457255 ) ) ;
#4406=DIRECTION ( 'NONE',  ( 2.220446049250313081E-16, 0.7071067811865452413, 0.7071067811865497932 ) ) ;
#4431=ORIENTED_EDGE ( 'NONE', *, *, #15127, .F. ) ;
#4437=DIRECTION ( 'NONE',  ( 1.000000000000000000, -7.410738689372937262E-15, 7.410738689372897819E-15 ) ) ;
#4439=LINE ( 'NONE', #1688, #10202 ) ;
#4460=DIRECTION ( 'NONE',  ( 0.000000000000000000, -0.7071067811865493491, 0.7071067811865457964 ) ) ;
#4486=EDGE_CURVE ( 'NONE', #895, #11055, #10752, .T. ) ;
#4525=DIRECTION ( 'NONE',  ( -0.000000000000000000, -0.7071067811865456854, -0.7071067811865494601 ) ) ;
#4530=DIRECTION ( 'NONE',  ( 1.047444401652940007E-14, 0.7071067811865495711, -0.7071067811865454633 ) ) ;
#4538=DIRECTION ( 'NONE',  ( -0.7071067811865463515, 0.5000000000000023315, -0.4999999999999994449 ) ) ;
#4556=ADVANCED_FACE ( 'NONE', ( #843 ), #12793, .F. ) ;
#4562=VECTOR ( 'NONE', #4633, 1000.000000000000114 ) ;
#4571=EDGE_CURVE ( 'NONE', #5689, #3132, #5949, .T. ) ;
#4575=DIRECTION ( 'NONE',  ( -0.000000000000000000, -0.7071067811865456854, -0.7071067811865493491 ) ) ;
#4618=B_SPLINE_CURVE_WITH_KNOTS ( 'NONE', 3,
 ( #11544, #11357, #6776, #15790 ),
 .UNSPECIFIED., .F., .F.,
 ( 4, 4 ),
 ( 0.000000000000000000, 1.000000000000000000 ),
 .UNSPECIFIED. ) ;
#4633=DIRECTION ( 'NONE',  ( -2.775557561562890858E-16, 0.7071067811865456854, 0.7071067811865493491 ) ) ;
#4634=CARTESIAN_POINT ( 'NONE',  ( -0.04166183285594760033, 33.84354264162095660, 52.64110397985704282 ) ) ;
#4639=DIRECTION ( 'NONE',  ( -0.000000000000000000, 0.7071067811865497932, -0.7071067811865452413 ) ) ;
#4666=LINE ( 'NONE', #10623, #1325 ) ;
#4717=ORIENTED_EDGE ( 'NONE', *, *, #1092, .T. ) ;
#4721=VECTOR ( 'NONE', #13894, 1000.000000000000000 ) ;
#4732=DIRECTION ( 'NONE',  ( -2.775557561562883462E-16, 0.7071067811865454633, 0.7071067811865495711 ) ) ;
#4733=CARTESIAN_POINT ( 'NONE',  ( -0.08332366571188480620, 33.84322526524066177, 52.64078660347674798 ) ) ;
#4737=VECTOR ( 'NONE', #17814, 1000.000000000000000 ) ;
#4738=CARTESIAN_POINT ( 'NONE',  ( -4.042620306204127267, 26.80012125920696064, 59.68389060951041358 ) ) ;
#4763=AXIS2_PLACEMENT_3D ( 'NONE', #7503, #1432, #7407 ) ;
#4764=EDGE_CURVE ( 'NONE', #4322, #12056, #7186, .T. ) ;
#4769=ORIENTED_EDGE ( 'NONE', *, *, #10982, .T. ) ;
#4791=EDGE_LOOP ( 'NONE', ( #3708, #3844, #17141, #5446, #1051 ) ) ;
#4805=ORIENTED_EDGE ( 'NONE', *, *, #13073, .T. ) ;
#4807=DIRECTION ( 'NONE',  ( 0.7071067811865414665, -0.5000000000000057732, 0.5000000000000028866 ) ) ;
#4815=DIRECTION ( 'NONE',  ( 0.000000000000000000, 0.000000000000000000, 1.000000000000000000 ) ) ;
#4827=DIRECTION ( 'NONE',  ( -0.000000000000000000, 0.7071067811865497932, -0.7071067811865452413 ) ) ;
#4847=CARTESIAN_POINT ( 'NONE',  ( -0.1250000000000104083, 27.16170093578836031, 58.97002704785691662 ) ) ;
#4851=AXIS2_PLACEMENT_3D ( 'NONE', #6420, #12582, #18576 ) ;
#4855=SURFACE_STYLE_USAGE ( .BOTH. , #12294 ) ;
#4868=PLANE ( 'NONE',  #15624 ) ;
#4891=ORIENTED_EDGE ( 'NONE', *, *, #1564, .F. ) ;
#4898=CARTESIAN_POINT ( 'NONE',  ( -2.492551403682614186, 28.10514068711927749, 58.38014068711927251 ) ) ;
#4907=EDGE_LOOP ( 'NONE', ( #2823, #14575, #18369, #4127, #15491 ) ) ;
#4914=LINE ( 'NONE', #9404, #15959 ) ;
#4925=DIRECTION ( 'NONE',  ( -0.000000000000000000, 0.7071067811865493491, -0.7071067811865456854 ) ) ;
#4953=LINE ( 'NONE', #15436, #15475 ) ;
#4954=PRESENTATION_STYLE_ASSIGNMENT (( #4855 ) ) ;
#4974=AXIS2_PLACEMENT_3D ( 'NONE', #16134, #11418, #8305 ) ;
#5015=DIRECTION ( 'NONE',  ( 0.000000000000000000, -0.7071067811865457964, -0.7071067811865492381 ) ) ;
#5023=DIRECTION ( 'NONE',  ( 1.110223024625156540E-16, 0.7071067811865455743, 0.7071067811865494601 ) ) ;
#5031=ORIENTED_EDGE ( 'NONE', *, *, #11769, .T. ) ;
#5039=ORIENTED_EDGE ( 'NONE', *, *, #9036, .T. ) ;
#5051=EDGE_LOOP ( 'NONE', ( #881, #11264, #6472, #779 ) ) ;
#5052=EDGE_CURVE ( 'NONE', #17270, #9938, #13728, .T. ) ;
#5061=EDGE_CURVE ( 'NONE', #6083, #9185, #6487, .T. ) ;
#5092=CARTESIAN_POINT ( 'NONE',  ( 4.012830983233651061, 32.52836399182262994, 53.60336399182268252 ) ) ;
#5103=ORIENTED_EDGE ( 'NONE', *, *, #5061, .F. ) ;
#5105=EDGE_LOOP ( 'NONE', ( #5985, #18335, #3220, #12115 ) ) ;
#5145=UNCERTAINTY_MEASURE_WITH_UNIT (LENGTH_MEASURE( 1.000000000000000082E-05 ), #3280, 'distance_accuracy_value', 'NONE');
#5181=EDGE_CURVE ( 'NONE', #7943, #13315, #14396, .T. ) ;
#5197=CARTESIAN_POINT ( 'NONE',  ( 2.492551403682558675, 27.92836399182260720, 58.20336399182267684 ) ) ;
#5199=DIRECTION ( 'NONE',  ( -0.000000000000000000, 0.7071067811865456854, 0.7071067811865493491 ) ) ;
#5200=VERTEX_POINT ( 'NONE', #2261 ) ;
#5206=FACE_OUTER_BOUND ( 'NONE', #4400, .T. ) ;
#5229=CARTESIAN_POINT ( 'NONE',  ( -0.1250000000000104083, 33.66708332270461312, 52.46464466094069934 ) ) ;
#5268=CARTESIAN_POINT ( 'NONE',  ( -1.040834085586084257E-14, 29.74264068711926257, 56.74264068711929809 ) ) ;
#5320=CARTESIAN_POINT ( 'NONE',  ( -4.012830983233618198, 32.52836399182267257, 53.60336399182263989 ) ) ;
#5327=CARTESIAN_POINT ( 'NONE',  ( -4.012830983233701687, 26.60336399182265055, 59.52836399182262994 ) ) ;
#5357=( NAMED_UNIT ( * ) PLANE_ANGLE_UNIT ( ) SI_UNIT ( $, .RADIAN. ) );
#5364=EDGE_LOOP ( 'NONE', ( #10754, #13809, #2711, #9469, #12213, #7654, #3655, #2400, #2819, #2556, #1072, #15373, #4150, #9302, #16672 ) ) ;
#5375=DIRECTION ( 'NONE',  ( -0.000000000000000000, 0.7071067811865452413, 0.7071067811865497932 ) ) ;
#5393=CARTESIAN_POINT ( 'NONE',  ( -4.189607678530337331, 26.72836399182265055, 59.40336399182262284 ) ) ;
#5394=ORIENTED_EDGE ( 'NONE', *, *, #11769, .F. ) ;
#5395=PLANE ( 'NONE',  #8802 ) ;
#5407=ORIENTED_EDGE ( 'NONE', *, *, #9343, .T. ) ;
#5420=ADVANCED_FACE ( 'NONE', ( #10159 ), #16159, .T. ) ;
#5425=LINE ( 'NONE', #11382, #12086 ) ;
#5426=ORIENTED_EDGE ( 'NONE', *, *, #14108, .T. ) ;
#5433=PLANE ( 'NONE',  #6588 ) ;
#5435=ADVANCED_FACE ( 'NONE', ( #3517 ), #6367, .T. ) ;
#5436=DIRECTION ( 'NONE',  ( -1.000000000000000000, 0.000000000000000000, -0.000000000000000000 ) ) ;
#5438=LINE ( 'NONE', #12874, #13411 ) ;
#5439=DIRECTION ( 'NONE',  ( -0.7071067811865487940, -0.5000000000000003331, 0.4999999999999979461 ) ) ;
#5446=ORIENTED_EDGE ( 'NONE', *, *, #2495, .F. ) ;
#5453=ORIENTED_EDGE ( 'NONE', *, *, #1812, .T. ) ;
#5476=CARTESIAN_POINT ( 'NONE',  ( -4.101219330881938241, 32.64264068711930378, 53.84264068711927109 ) ) ;
#5478=CARTESIAN_POINT ( 'NONE',  ( -1.040834085586084257E-14, 30.30832611206852079, 47.69167388793148632 ) ) ;
#5479=VERTEX_POINT ( 'NONE', #14094 ) ;
#5489=CARTESIAN_POINT ( 'NONE',  ( 0.1249999999999895917, 33.66708332270461312, 52.46464466094069934 ) ) ;
#5491=ORIENTED_EDGE ( 'NONE', *, *, #7649, .T. ) ;
#5497=ORIENTED_EDGE ( 'NONE', *, *, #17416, .F. ) ;
#5499=VECTOR ( 'NONE', #4538, 1000.000000000000000 ) ;
#5505=LINE ( 'NONE', #6793, #13292 ) ;
#5541=EDGE_CURVE ( 'NONE', #17455, #5479, #10134, .T. ) ;
#5563=VERTEX_POINT ( 'NONE', #14658 ) ;
#5622=DIRECTION ( 'NONE',  ( 2.665111688417744333E-15, 1.000000000000000000, 0.000000000000000000 ) ) ;
#5635=AXIS2_PLACEMENT_3D ( 'NONE', #14907, #9213, #15106 ) ;
#5673=ORIENTED_EDGE ( 'NONE', *, *, #14059, .T. ) ;
#5684=AXIS2_PLACEMENT_3D ( 'NONE', #15850, #9768, #12798 ) ;
#5689=VERTEX_POINT ( 'NONE', #10534 ) ;
#5709=CARTESIAN_POINT ( 'NONE',  ( -0.08838834764833032598, 29.80514068711926612, 56.68014068711929809 ) ) ;
#5728=DIRECTION ( 'NONE',  ( 0.000000000000000000, 0.7071067811865456854, 0.7071067811865494601 ) ) ;
#5733=CARTESIAN_POINT ( 'NONE',  ( -5.799326430397251819, 29.65377616443625541, 56.83055285973284754 ) ) ;
#5763=VERTEX_POINT ( 'NONE', #17178 ) ;
#5764=VERTEX_POINT ( 'NONE', #9983 ) ;
#5786=VERTEX_POINT ( 'NONE', #889 ) ;
#5788=EDGE_CURVE ( 'NONE', #16741, #2080, #8814, .T. ) ;
#5807=ORIENTED_EDGE ( 'NONE', *, *, #3607, .T. ) ;
#5813=CARTESIAN_POINT ( 'NONE',  ( 0.08332044287238019042, 25.64046917798804515, 60.84354269072931487 ) ) ;
#5814=EDGE_CURVE ( 'NONE', #12801, #9275, #14079, .T. ) ;
#5819=ORIENTED_EDGE ( 'NONE', *, *, #2657, .F. ) ;
#5852=VECTOR ( 'NONE', #17395, 1000.000000000000000 ) ;
#5869=DIRECTION ( 'NONE',  ( 0.000000000000000000, -0.7071067811865493491, 0.7071067811865457964 ) ) ;
#5874=DIRECTION ( 'NONE',  ( 0.000000000000000000, 0.7071067811865456854, 0.7071067811865494601 ) ) ;
#5878=VERTEX_POINT ( 'NONE', #1378 ) ;
#5903=CARTESIAN_POINT ( 'NONE',  ( 2.492551403682577771, 31.20336399182262710, 54.92836399182266405 ) ) ;
#5941=DIRECTION ( 'NONE',  ( -2.775557561562890858E-16, 0.7071067811865456854, 0.7071067811865493491 ) ) ;
#5942=VECTOR ( 'NONE', #17632, 1000.000000000000000 ) ;
#5949=CIRCLE ( 'NONE', #18183, 5.800000000000007816 ) ;
#5950=PLANE ( 'NONE',  #18036 ) ;
#5967=VERTEX_POINT ( 'NONE', #14906 ) ;
#5985=ORIENTED_EDGE ( 'NONE', *, *, #11656, .F. ) ;
#5995=CYLINDRICAL_SURFACE ( 'NONE', #19129, 6.799999999999997158 ) ;
#5999=EDGE_LOOP ( 'NONE', ( #12053, #10256, #5426, #5497, #13808 ) ) ;
#6013=EDGE_CURVE ( 'NONE', #5200, #2690, #8716, .T. ) ;
#6016=B_SPLINE_CURVE_WITH_KNOTS ( 'NONE', 3,
 ( #10726, #17797, #16328, #2895 ),
 .UNSPECIFIED., .F., .F.,
 ( 4, 4 ),
 ( 0.000000000000000000, 1.000000000000000000 ),
 .UNSPECIFIED. ) ;
#6022=ORIENTED_EDGE ( 'NONE', *, *, #15854, .F. ) ;
#6034=PLANE ( 'NONE',  #4370 ) ;
#6047=CARTESIAN_POINT ( 'NONE',  ( -4.189131392896629613, 26.90500129688593134, 59.57932772728315030 ) ) ;
#6051=CARTESIAN_POINT ( 'NONE',  ( 0.1249999999999895917, 33.84290755733280065, 52.64142146683631296 ) ) ;
#6057=ORIENTED_EDGE ( 'NONE', *, *, #3312, .F. ) ;
#6075=DIRECTION ( 'NONE',  ( -1.047444401652940007E-14, -0.7071067811865495711, 0.7071067811865454633 ) ) ;
#6079=ORIENTED_EDGE ( 'NONE', *, *, #6730, .T. ) ;
#6083=VERTEX_POINT ( 'NONE', #11318 ) ;
#6094=VERTEX_POINT ( 'NONE', #17126 ) ;
#6098=CARTESIAN_POINT ( 'NONE',  ( 5.799999999999985612, 29.65425233947092920, 56.47747564417436195 ) ) ;
#6119=DIRECTION ( 'NONE',  ( -1.000000000000000000, 2.470246229790980797E-15, -2.470246229790967386E-15 ) ) ;
#6137=ADVANCED_FACE ( 'NONE', ( #11600 ), #6034, .T. ) ;
#6159=PRODUCT_DEFINITION_SHAPE ( 'NONE', 'NONE',  #7639 ) ;
#6175=EDGE_CURVE ( 'NONE', #1607, #3132, #12795, .T. ) ;
#6198=EDGE_LOOP ( 'NONE', ( #12639, #14500, #12662, #7559 ) ) ;
#6246=ORIENTED_EDGE ( 'NONE', *, *, #8922, .F. ) ;
#6253=CARTESIAN_POINT ( 'NONE',  ( -2.492551403682614186, 27.92836399182264273, 58.20336399182264131 ) ) ;
#6259=ORIENTED_EDGE ( 'NONE', *, *, #10599, .T. ) ;
#6277=ORIENTED_EDGE ( 'NONE', *, *, #1714, .T. ) ;
#6285=EDGE_CURVE ( 'NONE', #11383, #7718, #7888, .T. ) ;
#6300=VECTOR ( 'NONE', #5439, 1000.000000000000000 ) ;
#6309=EDGE_CURVE ( 'NONE', #9861, #9708, #1700, .T. ) ;
#6312=DIRECTION ( 'NONE',  ( 1.000000000000000000, 0.000000000000000000, 0.000000000000000000 ) ) ;
#6336=EDGE_CURVE ( 'NONE', #13749, #9185, #1801, .T. ) ;
#6338=LINE ( 'NONE', #3086, #16597 ) ;
#6350=ADVANCED_FACE ( 'NONE', ( #10711 ), #6413, .T. ) ;
#6356=ORIENTED_EDGE ( 'NONE', *, *, #12943, .F. ) ;
#6367=PLANE ( 'NONE',  #8127 ) ;
#6398=CARTESIAN_POINT ( 'NONE',  ( -4.042620306204046443, 32.68389060951044911, 53.80012125920694643 ) ) ;
#6412=ORIENTED_EDGE ( 'NONE', *, *, #1360, .F. ) ;
#6413=PLANE ( 'NONE',  #8732 ) ;
#6420=CARTESIAN_POINT ( 'NONE',  ( -1.040834085586084257E-14, 29.74264068711926257, 56.74264068711929809 ) ) ;
#6444=ORIENTED_EDGE ( 'NONE', *, *, #7742, .T. ) ;
#6472=ORIENTED_EDGE ( 'NONE', *, *, #4486, .F. ) ;
#6487=LINE ( 'NONE', #18352, #12527 ) ;
#6510=DIRECTION ( 'NONE',  ( 1.000000000000000000, -7.210288835911348201E-15, 7.602811950582247805E-15 ) ) ;
#6513=FACE_OUTER_BOUND ( 'NONE', #12126, .T. ) ;
#6529=DIRECTION ( 'NONE',  ( 0.000000000000000000, -0.7071067811865493491, 0.7071067811865457964 ) ) ;
#6535=CARTESIAN_POINT ( 'NONE',  ( 3.399999999999996803, 29.47747564417430155, 56.65425233947098604 ) ) ;
#6554=AXIS2_PLACEMENT_3D ( 'NONE', #14639, #18353, #10510 ) ;
#6570=VERTEX_POINT ( 'NONE', #2373 ) ;
#6579=AXIS2_PLACEMENT_3D ( 'NONE', #12751, #17273, #3839 ) ;
#6588=AXIS2_PLACEMENT_3D ( 'NONE', #18765, #914, #5622 ) ;
#6614=PLANE ( 'NONE',  #4851 ) ;
#6630=CARTESIAN_POINT ( 'NONE',  ( -1.040834085586084257E-14, 29.74264068711925901, 56.74264068711929809 ) ) ;
#6633=DIRECTION ( 'NONE',  ( 0.7071067811865561215, 0.4999999999999953926, -0.4999999999999925060 ) ) ;
#6638=CARTESIAN_POINT ( 'NONE',  ( -0.1250000000000104083, 27.16170093578836031, 58.97002704785691662 ) ) ;
#6659=CARTESIAN_POINT ( 'NONE',  ( 0.1249999999999895917, 25.46464466094064250, 60.66708332270462734 ) ) ;
#6677=DIRECTION ( 'NONE',  ( 0.000000000000000000, -0.7071067811865457964, -0.7071067811865492381 ) ) ;
#6686=CARTESIAN_POINT ( 'NONE',  ( 2.492551403682577771, 31.20336399182262710, 54.92836399182266405 ) ) ;
#6689=DIRECTION ( 'NONE',  ( 0.7071067811865512365, 0.4999999999999988898, -0.4999999999999959477 ) ) ;
#6722=CARTESIAN_POINT ( 'NONE',  ( -0.1250000000000104083, 33.66708332270461312, 52.46464466094069934 ) ) ;
#6730=EDGE_CURVE ( 'NONE', #576, #8618, #8724, .T. ) ;
#6770=VECTOR ( 'NONE', #7641, 1000.000000000000114 ) ;
#6775=DIRECTION ( 'NONE',  ( -1.000000000000000000, 7.210288835911348201E-15, -7.602811950582247805E-15 ) ) ;
#6776=CARTESIAN_POINT ( 'NONE',  ( -0.08332044287239959157, 25.64046917798804515, 60.84354269072931487 ) ) ;
#6777=ORIENTED_EDGE ( 'NONE', *, *, #12943, .T. ) ;
#6793=CARTESIAN_POINT ( 'NONE',  ( -5.800000000000006928, 29.47747564417435484, 56.65425233947093631 ) ) ;
#6817=SURFACE_SIDE_STYLE ('',( #835 ) ) ;
#6831=CARTESIAN_POINT ( 'NONE',  ( 2.492551403682558675, 27.92836399182260720, 58.20336399182267684 ) ) ;
#6841=CARTESIAN_POINT ( 'NONE',  ( 5.799999999999984723, 29.74264068711924835, 56.74264068711931230 ) ) ;
#6847=ORIENTED_EDGE ( 'NONE', *, *, #4486, .T. ) ;
#6849=ORIENTED_EDGE ( 'NONE', *, *, #7767, .F. ) ;
#6858=DIRECTION ( 'NONE',  ( -0.000000000000000000, 0.7071067811865456854, 0.7071067811865493491 ) ) ;
#6878=CARTESIAN_POINT ( 'NONE',  ( 0.1249999999999895917, 33.66708332270461312, 52.46464466094069934 ) ) ;
#6901=CIRCLE ( 'NONE', #17868, 5.800000000000007816 ) ;
#6903=LINE ( 'NONE', #12875, #6300 ) ;
#6923=VECTOR ( 'NONE', #17959, 1000.000000000000114 ) ;
#6932=ORIENTED_EDGE ( 'NONE', *, *, #15362, .T. ) ;
#6944=ORIENTED_EDGE ( 'NONE', *, *, #6730, .F. ) ;
#6960=EDGE_CURVE ( 'NONE', #5689, #14223, #15075, .T. ) ;
#6965=CARTESIAN_POINT ( 'NONE',  ( -5.800448907431086987, 29.68308948419218041, 56.80092238452520803 ) ) ;
#6995=DIRECTION ( 'NONE',  ( -2.220446049250312588E-16, 0.7071067811865453523, 0.7071067811865496822 ) ) ;
#7014=CARTESIAN_POINT ( 'NONE',  ( 3.399999999999996803, 29.47747564417430155, 56.65425233947098604 ) ) ;
#7069=LINE ( 'NONE', #6878, #7680 ) ;
#7089=EDGE_CURVE ( 'NONE', #16934, #5764, #6903, .T. ) ;
#7120=ORIENTED_EDGE ( 'NONE', *, *, #314, .F. ) ;
#7122=EDGE_CURVE ( 'NONE', #16368, #6094, #17978, .T. ) ;
#7157=VECTOR ( 'NONE', #10778, 1000.000000000000000 ) ;
#7186=LINE ( 'NONE', #12964, #12211 ) ;
#7187=FACE_OUTER_BOUND ( 'NONE', #18728, .T. ) ;
#7212=DIRECTION ( 'NONE',  ( 0.5773502691896335026, 0.8164965809277204833, 0.000000000000000000 ) ) ;
#7236=CARTESIAN_POINT ( 'NONE',  ( -2.315774708385926139, 31.32836399182264842, 54.80336399182263563 ) ) ;
#7252=EDGE_LOOP ( 'NONE', ( #4194, #5394, #15586, #4365 ) ) ;
#7264=CARTESIAN_POINT ( 'NONE',  ( 3.399999999999996803, 29.65425233947093631, 56.83102903476762435 ) ) ;
#7268=PLANE ( 'NONE',  #18651 ) ;
#7312=CARTESIAN_POINT ( 'NONE',  ( 5.799999999999985612, 29.47747564417429444, 56.65425233947099315 ) ) ;
#7357=LINE ( 'NONE', #7264, #13128 ) ;
#7407=DIRECTION ( 'NONE',  ( -0.000000000000000000, 0.000000000000000000, -1.000000000000000000 ) ) ;
#7421=EDGE_LOOP ( 'NONE', ( #415, #15199, #602, #4891 ) ) ;
#7434=CARTESIAN_POINT ( 'NONE',  ( -2.315774708385926139, 31.32836399182264842, 54.80336399182263563 ) ) ;
#7453=CARTESIAN_POINT ( 'NONE',  ( -1.040834085586084257E-14, 29.74264068711926257, 56.74264068711929809 ) ) ;
#7459=CARTESIAN_POINT ( 'NONE',  ( 5.799999999999985612, 29.47747564417429444, 56.65425233947099315 ) ) ;
#7503=CARTESIAN_POINT ( 'NONE',  ( -0.1250000000000104083, 25.46464466094064250, 60.66708332270462734 ) ) ;
#7504=VECTOR ( 'NONE', #11915, 1000.000000000000000 ) ;
#7508=CARTESIAN_POINT ( 'NONE',  ( 2.315774708385941683, 31.50514068711926541, 54.98014068711930236 ) ) ;
#7513=CARTESIAN_POINT ( 'NONE',  ( -4.012830983233701687, 26.60336399182265055, 59.52836399182262994 ) ) ;
#7528=ORIENTED_EDGE ( 'NONE', *, *, #4353, .F. ) ;
#7531=DIRECTION ( 'NONE',  ( 0.000000000000000000, 0.7071067811865452413, 0.7071067811865497932 ) ) ;
#7536=VECTOR ( 'NONE', #12560, 1000.000000000000000 ) ;
#7555=DIRECTION ( 'NONE',  ( 0.000000000000000000, 0.7071067811865493491, -0.7071067811865457964 ) ) ;
#7559=ORIENTED_EDGE ( 'NONE', *, *, #18383, .T. ) ;
#7578=CARTESIAN_POINT ( 'NONE',  ( 4.012354697599942455, 32.70432772728315740, 53.78000129688596331 ) ) ;
#7618=CARTESIAN_POINT ( 'NONE',  ( -1.040834085586084257E-14, 29.03553390593270578, 56.03553390593273775 ) ) ;
#7637=DIRECTION ( 'NONE',  ( -0.5773502691896360561, -0.8164965809277188180, 0.000000000000000000 ) ) ;
#7639=PRODUCT_DEFINITION ( 'UNKNOWN', '', #2355, #19042 ) ;
#7641=DIRECTION ( 'NONE',  ( 0.7071067811865389130, -0.5000000000000073275, 0.5000000000000048850 ) ) ;
#7642=EDGE_LOOP ( 'NONE', ( #16300, #11232, #3427, #3786, #12347 ) ) ;
#7646=DIRECTION ( 'NONE',  ( 1.000000000000000000, 0.000000000000000000, 0.000000000000000000 ) ) ;
#7649=EDGE_CURVE ( 'NONE', #2217, #1789, #8635, .T. ) ;
#7653=CARTESIAN_POINT ( 'NONE',  ( -2.492551403682565780, 31.38014068711928672, 55.10514068711927393 ) ) ;
#7654=ORIENTED_EDGE ( 'NONE', *, *, #9639, .F. ) ;
#7673=UNCERTAINTY_MEASURE_WITH_UNIT (LENGTH_MEASURE( 1.000000000000000082E-05 ), #15837, 'distance_accuracy_value', 'NONE');
#7680=VECTOR ( 'NONE', #12849, 1000.000000000000000 ) ;
#7688=CARTESIAN_POINT ( 'NONE',  ( 4.012830983233625304, 26.60336399182260791, 59.52836399182266547 ) ) ;
#7689=PLANE ( 'NONE',  #10363 ) ;
#7706=DIRECTION ( 'NONE',  ( -0.000000000000000000, -0.7071067811865493491, 0.7071067811865456854 ) ) ;
#7716=DIRECTION ( 'NONE',  ( -1.942890293094023946E-16, 0.7071067811865456854, 0.7071067811865494601 ) ) ;
#7718=VERTEX_POINT ( 'NONE', #10588 ) ;
#7738=DIRECTION ( 'NONE',  ( 2.220446049250312834E-16, 0.7071067811865455743, 0.7071067811865493491 ) ) ;
#7742=EDGE_CURVE ( 'NONE', #15997, #2343, #48, .T. ) ;
#7756=ORIENTED_EDGE ( 'NONE', *, *, #7122, .T. ) ;
#7767=EDGE_CURVE ( 'NONE', #9938, #16368, #11966, .T. ) ;
#7783=DIRECTION ( 'NONE',  ( -0.000000000000000000, 0.7071067811865452413, 0.7071067811865497932 ) ) ;
#7787=DIRECTION ( 'NONE',  ( 0.000000000000000000, -0.7071067811865495711, 0.7071067811865454633 ) ) ;
#7833=AXIS2_PLACEMENT_3D ( 'NONE', #3277, #527, #12475 ) ;
#7840=PLANE ( 'NONE',  #15392 ) ;
#7866=DIRECTION ( 'NONE',  ( -1.000000000000000000, 0.000000000000000000, 0.000000000000000000 ) ) ;
#7888=LINE ( 'NONE', #12380, #12196 ) ;
#7919=EDGE_LOOP ( 'NONE', ( #224, #181, #5453, #18333 ) ) ;
#7935=DIRECTION ( 'NONE',  ( -0.7071067811865486830, -0.5000000000000005551, 0.4999999999999978351 ) ) ;
#7942=ORIENTED_EDGE ( 'NONE', *, *, #11656, .T. ) ;
#7943=VERTEX_POINT ( 'NONE', #10780 ) ;
#7958=CARTESIAN_POINT ( 'NONE',  ( 0.1249999999999895917, 25.46464466094064250, 60.66708332270462734 ) ) ;
#7966=LINE ( 'NONE', #598, #7536 ) ;
#7974=ADVANCED_FACE ( 'NONE', ( #18427 ), #7840, .T. ) ;
#7989=FACE_OUTER_BOUND ( 'NONE', #10086, .T. ) ;
#7991=SURFACE_STYLE_FILL_AREA ( #13860 ) ;
#8037=CIRCLE ( 'NONE', #515, 6.799999999999999822 ) ;
#8048=CARTESIAN_POINT ( 'NONE',  ( 5.800448907431066559, 29.68308948419212712, 56.80092238452526487 ) ) ;
#8055=AXIS2_PLACEMENT_3D ( 'NONE', #18453, #5023, #10983 ) ;
#8065=DIRECTION ( 'NONE',  ( 2.775557561562890858E-16, 0.7071067811865454633, 0.7071067811865496822 ) ) ;
#8067=CARTESIAN_POINT ( 'NONE',  ( -4.101219330881938241, 32.64264068711930378, 53.84264068711927109 ) ) ;
#8083=ADVANCED_FACE ( 'NONE', ( #18986 ), #11419, .F. ) ;
#8103=DIRECTION ( 'NONE',  ( -2.775557561562890858E-16, 0.7071067811865454633, 0.7071067811865496822 ) ) ;
#8127=AXIS2_PLACEMENT_3D ( 'NONE', #5092, #7935, #9293 ) ;
#8147=CARTESIAN_POINT ( 'NONE',  ( -0.1250000000000104083, 33.84386001800125143, 52.64142135623733765 ) ) ;
#8152=CIRCLE ( 'NONE', #3459, 6.799999999999999822 ) ;
#8180=CIRCLE ( 'NONE', #38, 5.800000000000007816 ) ;
#8185=DIRECTION ( 'NONE',  ( 0.7071067811865561215, 0.4999999999999953926, -0.4999999999999925060 ) ) ;
#8199=CARTESIAN_POINT ( 'NONE',  ( -1.040834085586084257E-14, 29.74264068711925901, 56.74264068711929809 ) ) ;
#8203=CARTESIAN_POINT ( 'NONE',  ( -0.1250000000000104083, 33.84290755733280776, 52.64142146683631296 ) ) ;
#8246=ORIENTED_EDGE ( 'NONE', *, *, #15244, .F. ) ;
#8280=LINE ( 'NONE', #2578, #3444 ) ;
#8287=CARTESIAN_POINT ( 'NONE',  ( -5.799326430397249155, 29.83055285973289372, 56.65377616443620212 ) ) ;
#8290=LINE ( 'NONE', #6722, #17406 ) ;
#8292=VERTEX_POINT ( 'NONE', #7508 ) ;
#8294=( NAMED_UNIT ( * ) SI_UNIT ( $, .STERADIAN. ) SOLID_ANGLE_UNIT ( ) );
#8305=DIRECTION ( 'NONE',  ( -3.491481338843133355E-15, -0.7071067811865495711, 0.7071067811865454633 ) ) ;
#8311=DIRECTION ( 'NONE',  ( 2.220446049250313081E-16, 0.7071067811865452413, 0.7071067811865497932 ) ) ;
#8323=DIRECTION ( 'NONE',  ( 1.000000000000000000, 0.000000000000000000, 0.000000000000000000 ) ) ;
#8356=EDGE_CURVE ( 'NONE', #5200, #15466, #9449, .T. ) ;
#8375=FACE_OUTER_BOUND ( 'NONE', #12145, .T. ) ;
#8386=FACE_OUTER_BOUND ( 'NONE', #10408, .T. ) ;
#8417=DIRECTION ( 'NONE',  ( -0.000000000000000000, -0.7071067811865493491, 0.7071067811865456854 ) ) ;
#8428=ORIENTED_EDGE ( 'NONE', *, *, #44, .F. ) ;
#8443=ORIENTED_EDGE ( 'NONE', *, *, #15327, .F. ) ;
#8456=VECTOR ( 'NONE', #1061, 1000.000000000000114 ) ;
#8481=VECTOR ( 'NONE', #2236, 1000.000000000000227 ) ;
#8502=ORIENTED_EDGE ( 'NONE', *, *, #17427, .T. ) ;
#8514=LINE ( 'NONE', #15590, #8456 ) ;
#8519=EDGE_CURVE ( 'NONE', #1447, #7718, #15549, .T. ) ;
#8545=ADVANCED_FACE ( 'NONE', ( #9175 ), #15160, .T. ) ;
#8557=PLANE ( 'NONE',  #15674 ) ;
#8570=CARTESIAN_POINT ( 'NONE',  ( 4.130991513055717768, 26.86292658466335936, 59.62172003681460808 ) ) ;
#8599=VECTOR ( 'NONE', #7866, 1000.000000000000000 ) ;
#8600=CARTESIAN_POINT ( 'NONE',  ( 2.492551403682577771, 31.38014068711926541, 55.10514068711930236 ) ) ;
#8618=VERTEX_POINT ( 'NONE', #1297 ) ;
#8634=DIRECTION ( 'NONE',  ( -2.775557561562890858E-16, 0.7071067811865454633, 0.7071067811865496822 ) ) ;
#8635=LINE ( 'NONE', #5709, #15064 ) ;
#8650=LINE ( 'NONE', #14341, #9092 ) ;
#8678=FACE_OUTER_BOUND ( 'NONE', #6198, .T. ) ;
#8716=LINE ( 'NONE', #4320, #15023 ) ;
#8724=LINE ( 'NONE', #16183, #19120 ) ;
#8725=CARTESIAN_POINT ( 'NONE',  ( 3.399999999999998135, 29.83102903476756751, 56.65425233947098604 ) ) ;
#8732=AXIS2_PLACEMENT_3D ( 'NONE', #13854, #6510, #13751 ) ;
#8738=VECTOR ( 'NONE', #4807, 1000.000000000000000 ) ;
#8744=VERTEX_POINT ( 'NONE', #14823 ) ;
#8782=CARTESIAN_POINT ( 'NONE',  ( 0.1249999999999895917, 25.46464466094064250, 60.66708332270462734 ) ) ;
#8802=AXIS2_PLACEMENT_3D ( 'NONE', #19105, #13009, #872 ) ;
#8814=B_SPLINE_CURVE_WITH_KNOTS ( 'NONE', 3,
 ( #989, #6965, #12840, #17451 ),
 .UNSPECIFIED., .F., .F.,
 ( 4, 4 ),
 ( 0.000000000000000000, 1.000000000000000000 ),
 .UNSPECIFIED. ) ;
#8823=ORIENTED_EDGE ( 'NONE', *, *, #6285, .F. ) ;
#8840=CARTESIAN_POINT ( 'NONE',  ( -4.189607678530337331, 26.72836399182265055, 59.40336399182262284 ) ) ;
#8849=ORIENTED_EDGE ( 'NONE', *, *, #15513, .T. ) ;
#8859=DIRECTION ( 'NONE',  ( 2.220446049250313081E-16, 0.7071067811865452413, 0.7071067811865497932 ) ) ;
#8873=FACE_OUTER_BOUND ( 'NONE', #2382, .T. ) ;
#8877=FACE_OUTER_BOUND ( 'NONE', #3558, .T. ) ;
#8895=CARTESIAN_POINT ( 'NONE',  ( 4.012354697599916697, 26.78000129688588871, 59.70432772728319293 ) ) ;
#8914=ORIENTED_EDGE ( 'NONE', *, *, #17986, .T. ) ;
#8918=ORIENTED_EDGE ( 'NONE', *, *, #7122, .F. ) ;
#8922=EDGE_CURVE ( 'NONE', #16741, #7718, #17863, .T. ) ;
#8925=DIRECTION ( 'NONE',  ( 0.7071067811865388020, -0.5000000000000074385, 0.5000000000000046629 ) ) ;
#8926=LINE ( 'NONE', #1491, #15198 ) ;
#8937=VECTOR ( 'NONE', #6075, 1000.000000000000000 ) ;
#8945=ORIENTED_EDGE ( 'NONE', *, *, #12920, .T. ) ;
#8997=PLANE ( 'NONE',  #398 ) ;
#9000=CARTESIAN_POINT ( 'NONE',  ( 4.012830983233651061, 32.52836399182262994, 53.60336399182268252 ) ) ;
#9021=DIRECTION ( 'NONE',  ( 3.491481338843133355E-15, 0.7071067811865495711, -0.7071067811865454633 ) ) ;
#9036=EDGE_CURVE ( 'NONE', #17270, #18191, #7966, .T. ) ;
#9071=AXIS2_PLACEMENT_3D ( 'NONE', #11163, #11441, #17160 ) ;
#9080=CARTESIAN_POINT ( 'NONE',  ( -0.08838834764832756430, 29.68014068711926257, 56.80514068711929809 ) ) ;
#9082=FACE_OUTER_BOUND ( 'NONE', #14363, .T. ) ;
#9092=VECTOR ( 'NONE', #2767, 999.9999999999998863 ) ;
#9105=LINE ( 'NONE', #16759, #6770 ) ;
#9135=CARTESIAN_POINT ( 'NONE',  ( -4.101219330882018177, 26.84264068711928530, 59.64264068711926825 ) ) ;
#9169=DIRECTION ( 'NONE',  ( -0.7071067811865561215, -0.4999999999999953926, 0.4999999999999925060 ) ) ;
#9175=FACE_OUTER_BOUND ( 'NONE', #1256, .T. ) ;
#9185=VERTEX_POINT ( 'NONE', #1268 ) ;
#9192=ORIENTED_EDGE ( 'NONE', *, *, #7767, .T. ) ;
#9213=DIRECTION ( 'NONE',  ( 0.000000000000000000, -0.7071067811865493491, 0.7071067811865456854 ) ) ;
#9217=ORIENTED_EDGE ( 'NONE', *, *, #6013, .T. ) ;
#9233=EDGE_LOOP ( 'NONE', ( #13092, #4088, #9721, #12536 ) ) ;
#9251=VECTOR ( 'NONE', #9706, 1000.000000000000114 ) ;
#9266=CARTESIAN_POINT ( 'NONE',  ( -0.1250000000000104083, 33.66708332270461312, 52.46464466094069934 ) ) ;
#9270=DIRECTION ( 'NONE',  ( 0.7071067811865437980, -0.5000000000000044409, 0.5000000000000008882 ) ) ;
#9275=VERTEX_POINT ( 'NONE', #1068 ) ;
#9293=DIRECTION ( 'NONE',  ( 0.5773502691896255090, -0.8164965809277261455, 0.000000000000000000 ) ) ;
#9297=CARTESIAN_POINT ( 'NONE',  ( -9.575581032440641666E-15, 24.22720779386417078, 60.84386001800125143 ) ) ;
#9302=ORIENTED_EDGE ( 'NONE', *, *, #16594, .T. ) ;
#9313=ORIENTED_EDGE ( 'NONE', *, *, #11452, .T. ) ;
#9322=CARTESIAN_POINT ( 'NONE',  ( -1.171838675107511455E-14, 29.65425233947094341, 56.83102903476761014 ) ) ;
#9332=PLANE ( 'NONE',  #9988 ) ;
#9343=EDGE_CURVE ( 'NONE', #15802, #4327, #11285, .T. ) ;
#9344=CIRCLE ( 'NONE', #16565, 5.800000000000007816 ) ;
#9387=EDGE_CURVE ( 'NONE', #5878, #6083, #6901, .T. ) ;
#9404=CARTESIAN_POINT ( 'NONE',  ( 0.1249999999999895917, 33.66708332270461312, 52.46464466094069934 ) ) ;
#9443=( GEOMETRIC_REPRESENTATION_CONTEXT ( 3 ) GLOBAL_UNCERTAINTY_ASSIGNED_CONTEXT ( ( #5145 ) ) GLOBAL_UNIT_ASSIGNED_CONTEXT ( ( #3280, #10718, #12583 ) ) REPRESENTATION_CONTEXT ( 'NONE', 'WORKASPACE' ) );
#9449=CIRCLE ( 'NONE', #10371, 5.800000000000007816 ) ;
#9451=AXIS2_PLACEMENT_3D ( 'NONE', #1694, #13643, #8323 ) ;
#9465=DIRECTION ( 'NONE',  ( 0.000000000000000000, 0.7071067811865456854, 0.7071067811865494601 ) ) ;
#9469=ORIENTED_EDGE ( 'NONE', *, *, #15945, .T. ) ;
#9499=EDGE_CURVE ( 'NONE', #16765, #5967, #10266, .T. ) ;
#9502=ORIENTED_EDGE ( 'NONE', *, *, #16201, .T. ) ;
#9505=CARTESIAN_POINT ( 'NONE',  ( -2.315774708385978098, 27.98014068711927038, 58.50514068711927251 ) ) ;
#9560=LINE ( 'NONE', #6638, #15546 ) ;
#9598=EDGE_CURVE ( 'NONE', #18891, #3990, #10954, .T. ) ;
#9614=ORIENTED_EDGE ( 'NONE', *, *, #11078, .T. ) ;
#9632=DIRECTION ( 'NONE',  ( 2.220446049250312834E-16, 0.7071067811865455743, 0.7071067811865493491 ) ) ;
#9633=DIRECTION ( 'NONE',  ( -0.5773502691896228445, 0.8164965809277280329, 0.000000000000000000 ) ) ;
#9639=EDGE_CURVE ( 'NONE', #16741, #2217, #8180, .T. ) ;
#9669=CARTESIAN_POINT ( 'NONE',  ( -5.800000000000006928, 29.65425233947099315, 56.47747564417430510 ) ) ;
#9692=VECTOR ( 'NONE', #7783, 1000.000000000000000 ) ;
#9706=DIRECTION ( 'NONE',  ( 2.220446049250312834E-16, 0.7071067811865455743, 0.7071067811865493491 ) ) ;
#9708=VERTEX_POINT ( 'NONE', #9297 ) ;
#9721=ORIENTED_EDGE ( 'NONE', *, *, #17193, .T. ) ;
#9743=VECTOR ( 'NONE', #18983, 1000.000000000000000 ) ;
#9749=LINE ( 'NONE', #14257, #16549 ) ;
#9751=CARTESIAN_POINT ( 'NONE',  ( -1.040834085586084257E-14, 33.84386001800125143, 52.64142135623732344 ) ) ;
#9768=DIRECTION ( 'NONE',  ( 0.000000000000000000, 0.7071067811865456854, 0.7071067811865493491 ) ) ;
#9790=EDGE_CURVE ( 'NONE', #895, #16765, #1235, .T. ) ;
#9817=CARTESIAN_POINT ( 'NONE',  ( 5.799999999999985612, 29.47747564417429444, 56.65425233947099315 ) ) ;
#9819=ORIENTED_EDGE ( 'NONE', *, *, #15513, .F. ) ;
#9860=ORIENTED_EDGE ( 'NONE', *, *, #2220, .T. ) ;
#9861=VERTEX_POINT ( 'NONE', #14771 ) ;
#9865=VECTOR ( 'NONE', #1830, 1000.000000000000000 ) ;
#9890=VERTEX_POINT ( 'NONE', #16231 ) ;
#9912=DIRECTION ( 'NONE',  ( -2.775557561562890858E-16, 0.7071067811865454633, 0.7071067811865496822 ) ) ;
#9938=VERTEX_POINT ( 'NONE', #7312 ) ;
#9958=DIRECTION ( 'NONE',  ( -0.7071067811865463515, 0.5000000000000023315, -0.4999999999999994449 ) ) ;
#9975=AXIS2_PLACEMENT_3D ( 'NONE', #1163, #16160, #2826 ) ;
#9983=CARTESIAN_POINT ( 'NONE',  ( 2.315774708385941683, 31.32836399182263065, 54.80336399182266405 ) ) ;
#9988=AXIS2_PLACEMENT_3D ( 'NONE', #15322, #1901, #2371 ) ;
#10005=FACE_OUTER_BOUND ( 'NONE', #18842, .T. ) ;
#10018=CARTESIAN_POINT ( 'NONE',  ( 0.1249999999999895917, 33.66708332270461312, 52.46464466094069934 ) ) ;
#10021=CARTESIAN_POINT ( 'NONE',  ( 0.1249999999999895917, 25.64142146683625612, 60.84290755733282197 ) ) ;
#10043=FACE_OUTER_BOUND ( 'NONE', #12587, .T. ) ;
#10055=ORIENTED_EDGE ( 'NONE', *, *, #4571, .F. ) ;
#10071=DIRECTION ( 'NONE',  ( 0.7071067811865414665, -0.5000000000000058842, 0.5000000000000028866 ) ) ;
#10086=EDGE_LOOP ( 'NONE', ( #17755, #15728, #12130, #3980, #12907, #12436, #10867, #9860, #11936, #4717, #6079, #13523, #10958, #16484, #750, #18311, #6246, #18350, #5491, #17226, #18677, #12449, #13639, #7942, #11845, #10875, #1169, #12719, #2279, #14807, #7756, #13595 ) ) ;
#10100=DIRECTION ( 'NONE',  ( 0.000000000000000000, 0.7071067811865454633, 0.7071067811865496822 ) ) ;
#10124=DIRECTION ( 'NONE',  ( -0.5773502691896202910, 0.8164965809277299202, 0.000000000000000000 ) ) ;
#10129=MANIFOLD_SOLID_BREP ( 'CirPattern1', #88 ) ;
#10134=LINE ( 'NONE', #1231, #15318 ) ;
#10159=FACE_OUTER_BOUND ( 'NONE', #5105, .T. ) ;
#10177=ADVANCED_FACE ( 'NONE', ( #1708 ), #7689, .F. ) ;
#10181=EDGE_CURVE ( 'NONE', #1809, #18891, #12947, .T. ) ;
#10202=VECTOR ( 'NONE', #4639, 1000.000000000000000 ) ;
#10256=ORIENTED_EDGE ( 'NONE', *, *, #5541, .T. ) ;
#10266=LINE ( 'NONE', #2929, #19108 ) ;
#10305=ORIENTED_EDGE ( 'NONE', *, *, #8519, .F. ) ;
#10306=VECTOR ( 'NONE', #237, 999.9999999999998863 ) ;
#10363=AXIS2_PLACEMENT_3D ( 'NONE', #13656, #239, #9633 ) ;
#10371=AXIS2_PLACEMENT_3D ( 'NONE', #13276, #9465, #10927 ) ;
#10384=FACE_OUTER_BOUND ( 'NONE', #12119, .T. ) ;
#10392=DIRECTION ( 'NONE',  ( -0.5773502691896282846, -0.8164965809277242581, 0.000000000000000000 ) ) ;
#10401=ORIENTED_EDGE ( 'NONE', *, *, #18600, .F. ) ;
#10408=EDGE_LOOP ( 'NONE', ( #9313, #2093, #1486, #15575 ) ) ;
#10420=EDGE_CURVE ( 'NONE', #17455, #5786, #2067, .T. ) ;
#10431=DIRECTION ( 'NONE',  ( 1.000000000000000000, -7.160938508832259686E-15, 7.660538869913580129E-15 ) ) ;
#10440=VECTOR ( 'NONE', #8859, 1000.000000000000000 ) ;
#10464=ADVANCED_FACE ( 'NONE', ( #16062 ), #5395, .T. ) ;
#10467=CARTESIAN_POINT ( 'NONE',  ( -3.400000000000017675, 29.65425233947097183, 56.47747564417432642 ) ) ;
#10469=VERTEX_POINT ( 'NONE', #4007 ) ;
#10485=DIRECTION ( 'NONE',  ( -0.000000000000000000, 0.000000000000000000, 1.000000000000000000 ) ) ;
#10510=DIRECTION ( 'NONE',  ( 0.000000000000000000, -0.7071067811865493491, 0.7071067811865457964 ) ) ;
#10516=LINE ( 'NONE', #7688, #10440 ) ;
#10534=CARTESIAN_POINT ( 'NONE',  ( 5.799326430397230503, 29.83055285973283333, 56.65377616443626607 ) ) ;
#10549=ORIENTED_EDGE ( 'NONE', *, *, #10931, .T. ) ;
#10573=ORIENTED_EDGE ( 'NONE', *, *, #9036, .F. ) ;
#10588=CARTESIAN_POINT ( 'NONE',  ( -3.400000000000020783, 29.65425233947096118, 56.83102903476758883 ) ) ;
#10599=EDGE_CURVE ( 'NONE', #19340, #5563, #13210, .T. ) ;
#10623=CARTESIAN_POINT ( 'NONE',  ( -0.08838834764832678714, 29.80514068711926257, 56.68014068711929809 ) ) ;
#10645=ORIENTED_EDGE ( 'NONE', *, *, #2432, .F. ) ;
#10671=EDGE_LOOP ( 'NONE', ( #15096, #2662, #2607, #990 ) ) ;
#10711=FACE_OUTER_BOUND ( 'NONE', #4791, .T. ) ;
#10718=( NAMED_UNIT ( * ) PLANE_ANGLE_UNIT ( ) SI_UNIT ( $, .RADIAN. ) );
#10726=CARTESIAN_POINT ( 'NONE',  ( -9.120482147295685276E-15, 33.84386001800124433, 52.64142135623733054 ) ) ;
#10728=LINE ( 'NONE', #15250, #15184 ) ;
#10752=LINE ( 'NONE', #16657, #4721 ) ;
#10754=ORIENTED_EDGE ( 'NONE', *, *, #6309, .F. ) ;
#10775=EDGE_LOOP ( 'NONE', ( #8823, #10401, #1669, #2417 ) ) ;
#10778=DIRECTION ( 'NONE',  ( -3.491481338843133355E-15, -0.7071067811865495711, 0.7071067811865454633 ) ) ;
#10780=CARTESIAN_POINT ( 'NONE',  ( 4.012830983233625304, 26.60336399182260791, 59.52836399182266547 ) ) ;
#10821=ADVANCED_FACE ( 'NONE', ( #8386 ), #16035, .F. ) ;
#10822=CARTESIAN_POINT ( 'NONE',  ( 0.1249999999999895917, 31.97002704785689531, 54.16170093578840294 ) ) ;
#10825=CARTESIAN_POINT ( 'NONE',  ( -5.800000000000006928, 29.47747564417435484, 56.65425233947093631 ) ) ;
#10867=ORIENTED_EDGE ( 'NONE', *, *, #12015, .T. ) ;
#10875=ORIENTED_EDGE ( 'NONE', *, *, #44, .T. ) ;
#10889=CARTESIAN_POINT ( 'NONE',  ( 4.189607678530287593, 32.40336399182262284, 53.72836399182268252 ) ) ;
#10893=LINE ( 'NONE', #11085, #13983 ) ;
#10909=FILL_AREA_STYLE_COLOUR ( '', #671 ) ;
#10927=DIRECTION ( 'NONE',  ( 0.000000000000000000, -0.7071067811865493491, 0.7071067811865457964 ) ) ;
#10931=EDGE_CURVE ( 'NONE', #885, #9861, #11860, .T. ) ;
#10942=VECTOR ( 'NONE', #11389, 1000.000000000000000 ) ;
#10954=LINE ( 'NONE', #2043, #8481 ) ;
#10958=ORIENTED_EDGE ( 'NONE', *, *, #6013, .F. ) ;
#10972=VECTOR ( 'NONE', #4437, 1000.000000000000000 ) ;
#10979=LINE ( 'NONE', #18261, #8599 ) ;
#10982=EDGE_CURVE ( 'NONE', #9890, #1607, #17960, .T. ) ;
#10983=DIRECTION ( 'NONE',  ( 0.7071067811865463515, -0.5000000000000023315, 0.4999999999999994449 ) ) ;
#10986=CARTESIAN_POINT ( 'NONE',  ( -4.072081901468758147, 32.66337542264481186, 53.82127119883317334 ) ) ;
#11035=FILL_AREA_STYLE ('',( #17311 ) ) ;
#11045=CARTESIAN_POINT ( 'NONE',  ( -4.189607678530257395, 32.40336399182267257, 53.72836399182263278 ) ) ;
#11053=EDGE_LOOP ( 'NONE', ( #11276, #13784, #6277, #18376 ) ) ;
#11055=VERTEX_POINT ( 'NONE', #5197 ) ;
#11057=ORIENTED_EDGE ( 'NONE', *, *, #18383, .F. ) ;
#11070=ADVANCED_FACE ( 'NONE', ( #18719 ), #3714, .T. ) ;
#11078=EDGE_CURVE ( 'NONE', #2281, #16368, #1810, .T. ) ;
#11085=CARTESIAN_POINT ( 'NONE',  ( 2.315774708385922587, 27.98014068711924551, 58.50514068711930804 ) ) ;
#11119=LINE ( 'NONE', #357, #2447 ) ;
#11143=EDGE_CURVE ( 'NONE', #5764, #8292, #16699, .T. ) ;
#11163=CARTESIAN_POINT ( 'NONE',  ( 4.189607678530260948, 26.72836399182260791, 59.40336399182267257 ) ) ;
#11178=EDGE_CURVE ( 'NONE', #14286, #8292, #17429, .T. ) ;
#11194=DIRECTION ( 'NONE',  ( 0.000000000000000000, 0.7071067811865452413, 0.7071067811865497932 ) ) ;
#11207=CARTESIAN_POINT ( 'NONE',  ( -5.800000000000005151, 29.74264068711930520, 56.74264068711926257 ) ) ;
#11213=( LENGTH_UNIT ( ) NAMED_UNIT ( * ) SI_UNIT ( .MILLI., .METRE. ) );
#11232=ORIENTED_EDGE ( 'NONE', *, *, #1564, .T. ) ;
#11248=CARTESIAN_POINT ( 'NONE',  ( -4.160453206537114923, 32.60057016663805740, 53.88344170207933104 ) ) ;
#11262=LINE ( 'NONE', #6686, #9251 ) ;
#11264=ORIENTED_EDGE ( 'NONE', *, *, #17986, .F. ) ;
#11276=ORIENTED_EDGE ( 'NONE', *, *, #16802, .F. ) ;
#11285=B_SPLINE_CURVE_WITH_KNOTS ( 'NONE', 3,
 ( #14987, #93, #1562, #191 ),
 .UNSPECIFIED., .F., .F.,
 ( 4, 4 ),
 ( 0.000000000000000000, 1.000000000000000000 ),
 .UNSPECIFIED. ) ;
#11292=PLANE ( 'NONE',  #13641 ) ;
#11318=CARTESIAN_POINT ( 'NONE',  ( -0.1250000000000104083, 25.64142146683625612, 60.84290755733282197 ) ) ;
#11350=ORIENTED_EDGE ( 'NONE', *, *, #13073, .F. ) ;
#11357=CARTESIAN_POINT ( 'NONE',  ( -0.04165538583021200641, 25.64078660347668759, 60.84386001800125854 ) ) ;
#11382=CARTESIAN_POINT ( 'NONE',  ( -3.400000000000017675, 29.65425233947097183, 56.47747564417432642 ) ) ;
#11383=VERTEX_POINT ( 'NONE', #13793 ) ;
#11389=DIRECTION ( 'NONE',  ( 1.000000000000000000, 0.000000000000000000, 0.000000000000000000 ) ) ;
#11403=PRESENTATION_STYLE_ASSIGNMENT (( #12784 ) ) ;
#11418=DIRECTION ( 'NONE',  ( 2.775557561562891351E-16, 0.7071067811865454633, 0.7071067811865495711 ) ) ;
#11419=PLANE ( 'NONE',  #5684 ) ;
#11429=VECTOR ( 'NONE', #13391, 1000.000000000000227 ) ;
#11441=DIRECTION ( 'NONE',  ( -0.7071067811865437980, 0.5000000000000044409, -0.5000000000000008882 ) ) ;
#11445=PLANE ( 'NONE',  #19076 ) ;
#11452=EDGE_CURVE ( 'NONE', #9890, #8292, #4666, .T. ) ;
#11464=ORIENTED_EDGE ( 'NONE', *, *, #10420, .F. ) ;
#11472=EDGE_CURVE ( 'NONE', #15997, #18408, #6016, .T. ) ;
#11506=DIRECTION ( 'NONE',  ( 0.000000000000000000, 0.7071067811865493491, -0.7071067811865457964 ) ) ;
#11536=LINE ( 'NONE', #17533, #5942 ) ;
#11544=CARTESIAN_POINT ( 'NONE',  ( -1.040834085586084257E-14, 25.64142135623728080, 60.84386001800126564 ) ) ;
#11571=ADVANCED_FACE ( 'NONE', ( #2201 ), #18395, .T. ) ;
#11582=DIRECTION ( 'NONE',  ( -0.7071067811865562325, -0.4999999999999955036, 0.4999999999999924505 ) ) ;
#11592=DIRECTION ( 'NONE',  ( 0.7071067811865535679, 0.4999999999999971134, -0.4999999999999944489 ) ) ;
#11596=LINE ( 'NONE', #13464, #18373 ) ;
#11600=FACE_OUTER_BOUND ( 'NONE', #15906, .T. ) ;
#11614=VECTOR ( 'NONE', #14241, 1000.000000000000114 ) ;
#11636=CARTESIAN_POINT ( 'NONE',  ( -4.101219330882018177, 26.84264068711928530, 59.64264068711926825 ) ) ;
#11653=VERTEX_POINT ( 'NONE', #14634 ) ;
#11655=ADVANCED_FACE ( 'NONE', ( #12960 ), #5433, .T. ) ;
#11656=EDGE_CURVE ( 'NONE', #9185, #17434, #19050, .T. ) ;
#11663=FACE_OUTER_BOUND ( 'NONE', #17628, .T. ) ;
#11668=DIRECTION ( 'NONE',  ( 0.7071067811865535679, 0.4999999999999971134, -0.4999999999999944489 ) ) ;
#11678=CARTESIAN_POINT ( 'NONE',  ( 0.1249999999999895917, 25.64142146683625612, 60.84290755733282197 ) ) ;
#11730=ORIENTED_EDGE ( 'NONE', *, *, #5052, .F. ) ;
#11750=PLANE ( 'NONE',  #5635 ) ;
#11769=EDGE_CURVE ( 'NONE', #4322, #8618, #8280, .T. ) ;
#11781=VERTEX_POINT ( 'NONE', #2386 ) ;
#11794=CARTESIAN_POINT ( 'NONE',  ( -4.012830983233618198, 32.52836399182267257, 53.60336399182263989 ) ) ;
#11815=ADVANCED_FACE ( 'NONE', ( #12770 ), #231, .T. ) ;
#11831=ORIENTED_EDGE ( 'NONE', *, *, #217, .F. ) ;
#11845=ORIENTED_EDGE ( 'NONE', *, *, #12916, .F. ) ;
#11857=CARTESIAN_POINT ( 'NONE',  ( 4.189607678530287593, 32.40336399182262284, 53.72836399182268252 ) ) ;
#11858=AXIS2_PLACEMENT_3D ( 'NONE', #2774, #4357, #16309 ) ;
#11860=B_SPLINE_CURVE_WITH_KNOTS ( 'NONE', 3,
 ( #11678, #5813, #3063, #16598 ),
 .UNSPECIFIED., .F., .F.,
 ( 4, 4 ),
 ( 0.000000000000000000, 1.000000000000000000 ),
 .UNSPECIFIED. ) ;
#11884=CARTESIAN_POINT ( 'NONE',  ( 4.189131392896579875, 32.57932772728315740, 53.90500129688597042 ) ) ;
#11892=VECTOR ( 'NONE', #8417, 1000.000000000000000 ) ;
#11896=CARTESIAN_POINT ( 'NONE',  ( 4.189131392896553230, 26.90500129688588871, 59.57932772728319293 ) ) ;
#11915=DIRECTION ( 'NONE',  ( -1.000000000000000000, 0.000000000000000000, 0.000000000000000000 ) ) ;
#11921=DIRECTION ( 'NONE',  ( 0.000000000000000000, 0.7071067811865497932, -0.7071067811865452413 ) ) ;
#11936=ORIENTED_EDGE ( 'NONE', *, *, #12920, .F. ) ;
#11945=DIRECTION ( 'NONE',  ( 0.000000000000000000, -0.7071067811865493491, 0.7071067811865457964 ) ) ;
#11946=VECTOR ( 'NONE', #8103, 1000.000000000000114 ) ;
#11966=LINE ( 'NONE', #7459, #6923 ) ;
#11968=CARTESIAN_POINT ( 'NONE',  ( -4.072081901468836307, 26.82127119883319466, 59.66337542264477634 ) ) ;
#11985=LINE ( 'NONE', #17977, #12792 ) ;
#12002=CARTESIAN_POINT ( 'NONE',  ( -9.575581032440643243E-15, 24.93431457505072402, 61.55096679918780467 ) ) ;
#12014=ORIENTED_EDGE ( 'NONE', *, *, #16599, .T. ) ;
#12015=EDGE_CURVE ( 'NONE', #18408, #10469, #3270, .T. ) ;
#12029=COLOUR_RGB ( '', 0.72549020, 0.75294118, 0.79215686) ;
#12053=ORIENTED_EDGE ( 'NONE', *, *, #17919, .F. ) ;
#12056=VERTEX_POINT ( 'NONE', #716 ) ;
#12086=VECTOR ( 'NONE', #9912, 1000.000000000000114 ) ;
#12113=DIRECTION ( 'NONE',  ( -2.220446049250312588E-16, 0.7071067811865453523, 0.7071067811865496822 ) ) ;
#12115=ORIENTED_EDGE ( 'NONE', *, *, #17994, .T. ) ;
#12119=EDGE_LOOP ( 'NONE', ( #4431, #5807, #18626, #12149, #6444 ) ) ;
#12126=EDGE_LOOP ( 'NONE', ( #17182, #15580, #18215, #17360 ) ) ;
#12130=ORIENTED_EDGE ( 'NONE', *, *, #217, .T. ) ;
#12145=EDGE_LOOP ( 'NONE', ( #1097, #5673, #1176, #3462 ) ) ;
#12149=ORIENTED_EDGE ( 'NONE', *, *, #11472, .F. ) ;
#12159=ADVANCED_FACE ( 'NONE', ( #13748 ), #9332, .T. ) ;
#12196=VECTOR ( 'NONE', #3370, 1000.000000000000000 ) ;
#12211=VECTOR ( 'NONE', #14738, 999.9999999999998863 ) ;
#12213=ORIENTED_EDGE ( 'NONE', *, *, #4353, .T. ) ;
#12229=EDGE_LOOP ( 'NONE', ( #563, #9819, #10573, #9502 ) ) ;
#12238=ADVANCED_FACE ( 'NONE', ( #12663 ), #17557, .T. ) ;
#12281=EDGE_CURVE ( 'NONE', #1809, #12841, #4027, .T. ) ;
#12290=LINE ( 'NONE', #13953, #10306 ) ;
#12294=SURFACE_SIDE_STYLE ('',( #7991 ) ) ;
#12305=DIRECTION ( 'NONE',  ( 0.000000000000000000, 0.7071067811865456854, 0.7071067811865494601 ) ) ;
#12328=CARTESIAN_POINT ( 'NONE',  ( 0.08838834764831179913, 29.68014068711925901, 56.80514068711929809 ) ) ;
#12347=ORIENTED_EDGE ( 'NONE', *, *, #10982, .F. ) ;
#12380=CARTESIAN_POINT ( 'NONE',  ( -3.400000000000017675, 29.83102903476760659, 56.65425233947095762 ) ) ;
#12395=DIRECTION ( 'NONE',  ( 0.000000000000000000, 0.7071067811865456854, 0.7071067811865493491 ) ) ;
#12436=ORIENTED_EDGE ( 'NONE', *, *, #706, .T. ) ;
#12444=CARTESIAN_POINT ( 'NONE',  ( -2.492551403682565780, 31.20336399182265552, 54.92836399182263563 ) ) ;
#12449=ORIENTED_EDGE ( 'NONE', *, *, #9387, .T. ) ;
#12452=CARTESIAN_POINT ( 'NONE',  ( 0.1249999999999895917, 31.97002704785689531, 54.16170093578840294 ) ) ;
#12456=PLANE ( 'NONE',  #8055 ) ;
#12470=EDGE_CURVE ( 'NONE', #6094, #14223, #7357, .T. ) ;
#12475=DIRECTION ( 'NONE',  ( -0.7071067811865414665, 0.5000000000000057732, -0.5000000000000028866 ) ) ;
#12476=ADVANCED_FACE ( 'NONE', ( #11663 ), #14711, .F. ) ;
#12482=EDGE_LOOP ( 'NONE', ( #17523, #4065, #5031, #6944 ) ) ;
#12483=CIRCLE ( 'NONE', #6554, 5.800000000000007816 ) ;
#12488=B_SPLINE_CURVE_WITH_KNOTS ( 'NONE', 3,
 ( #11636, #4402, #1157, #4301 ),
 .UNSPECIFIED., .F., .F.,
 ( 4, 4 ),
 ( 0.000000000000000000, 1.000000000000000000 ),
 .UNSPECIFIED. ) ;
#12491=CARTESIAN_POINT ( 'NONE',  ( 2.315774708385922587, 27.80336399182260720, 58.32836399182267684 ) ) ;
#12494=CARTESIAN_POINT ( 'NONE',  ( 4.012830983233625304, 26.60336399182260791, 59.52836399182266547 ) ) ;
#12527=VECTOR ( 'NONE', #4925, 1000.000000000000114 ) ;
#12536=ORIENTED_EDGE ( 'NONE', *, *, #11143, .T. ) ;
#12560=DIRECTION ( 'NONE',  ( -1.000000000000000000, 2.720046410331633524E-15, -2.220446049250313081E-15 ) ) ;
#12582=DIRECTION ( 'NONE',  ( 0.000000000000000000, 0.7071067811865456854, 0.7071067811865493491 ) ) ;
#12583=( NAMED_UNIT ( * ) SI_UNIT ( $, .STERADIAN. ) SOLID_ANGLE_UNIT ( ) );
#12587=EDGE_LOOP ( 'NONE', ( #6777, #1191, #2035, #17424 ) ) ;
#12592=DIRECTION ( 'NONE',  ( 0.000000000000000000, 0.7071067811865493491, -0.7071067811865456854 ) ) ;
#12635=LINE ( 'NONE', #12444, #3765 ) ;
#12639=ORIENTED_EDGE ( 'NONE', *, *, #2549, .T. ) ;
#12640=LINE ( 'NONE', #8147, #11892 ) ;
#12643=ADVANCED_FACE ( 'NONE', ( #1973 ), #4390, .T. ) ;
#12662=ORIENTED_EDGE ( 'NONE', *, *, #10181, .F. ) ;
#12663=FACE_OUTER_BOUND ( 'NONE', #1375, .T. ) ;
#12674=ORIENTED_EDGE ( 'NONE', *, *, #6336, .T. ) ;
#12706=CARTESIAN_POINT ( 'NONE',  ( -1.040834085586084257E-14, 34.55096679918779756, 51.93431457505078441 ) ) ;
#12713=LINE ( 'NONE', #6831, #15532 ) ;
#12719=ORIENTED_EDGE ( 'NONE', *, *, #18839, .T. ) ;
#12741=CARTESIAN_POINT ( 'NONE',  ( 0.1249999999999895917, 25.46464466094064250, 60.66708332270462734 ) ) ;
#12751=CARTESIAN_POINT ( 'NONE',  ( -1.040834085586084257E-14, 25.49999999999998934, 52.50000000000000000 ) ) ;
#12754=CARTESIAN_POINT ( 'NONE',  ( -4.012830983233701687, 26.60336399182265055, 59.52836399182262994 ) ) ;
#12770=FACE_OUTER_BOUND ( 'NONE', #1692, .T. ) ;
#12772=DIRECTION ( 'NONE',  ( 1.047444401652940007E-14, 0.7071067811865495711, -0.7071067811865454633 ) ) ;
#12784=SURFACE_STYLE_USAGE ( .BOTH. , #6817 ) ;
#12792=VECTOR ( 'NONE', #15499, 1000.000000000000114 ) ;
#12793=PLANE ( 'NONE',  #14052 ) ;
#12795=B_SPLINE_CURVE_WITH_KNOTS ( 'NONE', 3,
 ( #13552, #19252, #2672, #11884 ),
 .UNSPECIFIED., .F., .F.,
 ( 4, 4 ),
 ( 0.000000000000000000, 1.000000000000000000 ),
 .UNSPECIFIED. ) ;
#12798=DIRECTION ( 'NONE',  ( 0.000000000000000000, -0.7071067811865493491, 0.7071067811865456854 ) ) ;
#12801=VERTEX_POINT ( 'NONE', #5478 ) ;
#12805=ORIENTED_EDGE ( 'NONE', *, *, #15127, .T. ) ;
#12810=ADVANCED_FACE ( 'NONE', ( #5206 ), #15688, .T. ) ;
#12840=CARTESIAN_POINT ( 'NONE',  ( -5.800448837981398320, 29.71286850494553278, 56.77177811653244532 ) ) ;
#12841=VERTEX_POINT ( 'NONE', #5393 ) ;
#12849=DIRECTION ( 'NONE',  ( -0.000000000000000000, -0.7071067811865493491, 0.7071067811865456854 ) ) ;
#12868=MECHANICAL_DESIGN_GEOMETRIC_PRESENTATION_REPRESENTATION('',(#3160),#9443);
#12874=CARTESIAN_POINT ( 'NONE',  ( -4.189607678530337331, 26.72836399182265055, 59.40336399182262284 ) ) ;
#12875=CARTESIAN_POINT ( 'NONE',  ( 4.012830983233651061, 32.52836399182262994, 53.60336399182268252 ) ) ;
#12885=( NAMED_UNIT ( * ) PLANE_ANGLE_UNIT ( ) SI_UNIT ( $, .RADIAN. ) );
#12901=ORIENTED_EDGE ( 'NONE', *, *, #16599, .F. ) ;
#12907=ORIENTED_EDGE ( 'NONE', *, *, #11452, .F. ) ;
#12916=EDGE_CURVE ( 'NONE', #885, #17434, #8514, .T. ) ;
#12920=EDGE_CURVE ( 'NONE', #2343, #11653, #12640, .T. ) ;
#12922=CARTESIAN_POINT ( 'NONE',  ( -3.400000000000017675, 29.47747564417433352, 56.65425233947095052 ) ) ;
#12943=EDGE_CURVE ( 'NONE', #17726, #9708, #8152, .T. ) ;
#12947=LINE ( 'NONE', #5327, #11614 ) ;
#12948=DIRECTION ( 'NONE',  ( 0.7071067811865535679, 0.4999999999999973355, -0.4999999999999940048 ) ) ;
#12949=PLANE ( 'NONE',  #1128 ) ;
#12950=ORIENTED_EDGE ( 'NONE', *, *, #12281, .T. ) ;
#12960=FACE_OUTER_BOUND ( 'NONE', #290, .T. ) ;
#12964=CARTESIAN_POINT ( 'NONE',  ( -2.315774708385926139, 31.32836399182264842, 54.80336399182263563 ) ) ;
#12981=CARTESIAN_POINT ( 'NONE',  ( -1.040834085586084257E-14, 29.74264068711925901, 56.74264068711929809 ) ) ;
#12985=CARTESIAN_POINT ( 'NONE',  ( -5.800000000000005151, 29.74264068711930520, 56.74264068711926257 ) ) ;
#13005=CARTESIAN_POINT ( 'NONE',  ( -4.189131392896543460, 32.57932772728320003, 53.90500129688591358 ) ) ;
#13009=DIRECTION ( 'NONE',  ( 0.7071067811865390240, -0.5000000000000073275, 0.5000000000000048850 ) ) ;
#13010=EDGE_CURVE ( 'NONE', #8618, #2690, #6338, .T. ) ;
#13020=EDGE_LOOP ( 'NONE', ( #14499, #2822, #97, #816 ) ) ;
#13073=EDGE_CURVE ( 'NONE', #89, #1447, #10728, .T. ) ;
#13076=LINE ( 'NONE', #7014, #16645 ) ;
#13092=ORIENTED_EDGE ( 'NONE', *, *, #11178, .F. ) ;
#13128=VECTOR ( 'NONE', #9021, 1000.000000000000000 ) ;
#13134=DIRECTION ( 'NONE',  ( 0.5773502691896176264, -0.8164965809277319186, 0.000000000000000000 ) ) ;
#13142=LINE ( 'NONE', #5903, #5499 ) ;
#13145=DIRECTION ( 'NONE',  ( 0.7071067811865486830, 0.5000000000000005551, -0.4999999999999978351 ) ) ;
#13161=PLANE ( 'NONE',  #11858 ) ;
#13178=VECTOR ( 'NONE', #5941, 1000.000000000000114 ) ;
#13186=VECTOR ( 'NONE', #9958, 1000.000000000000000 ) ;
#13210=LINE ( 'NONE', #9266, #2562 ) ;
#13213=EDGE_CURVE ( 'NONE', #89, #106, #18684, .T. ) ;
#13219=ORIENTED_EDGE ( 'NONE', *, *, #15264, .T. ) ;
#13235=FACE_OUTER_BOUND ( 'NONE', #17331, .T. ) ;
#13274=CARTESIAN_POINT ( 'NONE',  ( 5.799999999999984723, 29.74264068711924835, 56.74264068711931230 ) ) ;
#13276=CARTESIAN_POINT ( 'NONE',  ( -1.040834085586084257E-14, 29.74264068711925901, 56.74264068711929809 ) ) ;
#13291=AXIS2_PLACEMENT_3D ( 'NONE', #7434, #13402, #7637 ) ;
#13292=VECTOR ( 'NONE', #8634, 1000.000000000000114 ) ;
#13306=CARTESIAN_POINT ( 'NONE',  ( -1.040834085586084257E-14, 29.74264068711925901, 56.74264068711929809 ) ) ;
#13311=ORIENTED_EDGE ( 'NONE', *, *, #17882, .F. ) ;
#13315=VERTEX_POINT ( 'NONE', #12491 ) ;
#13363=ADVANCED_FACE ( 'NONE', ( #8375 ), #2772, .T. ) ;
#13377=CARTESIAN_POINT ( 'NONE',  ( -4.012354697599906928, 32.70432772728319293, 53.78000129688592068 ) ) ;
#13383=FACE_OUTER_BOUND ( 'NONE', #5999, .T. ) ;
#13391=DIRECTION ( 'NONE',  ( -2.220446049250312588E-16, 0.7071067811865453523, 0.7071067811865496822 ) ) ;
#13402=DIRECTION ( 'NONE',  ( -0.7071067811865390240, 0.5000000000000073275, -0.5000000000000048850 ) ) ;
#13411=VECTOR ( 'NONE', #6995, 1000.000000000000227 ) ;
#13423=FACE_OUTER_BOUND ( 'NONE', #7919, .T. ) ;
#13450=ORIENTED_EDGE ( 'NONE', *, *, #15362, .F. ) ;
#13461=B_SPLINE_CURVE_WITH_KNOTS ( 'NONE', 3,
 ( #13005, #11248, #4106, #5476 ),
 .UNSPECIFIED., .F., .F.,
 ( 4, 4 ),
 ( 0.000000000000000000, 1.000000000000000000 ),
 .UNSPECIFIED. ) ;
#13464=CARTESIAN_POINT ( 'NONE',  ( 3.399999999999996803, 29.65425233947092920, 56.47747564417434774 ) ) ;
#13483=LINE ( 'NONE', #3091, #7504 ) ;
#13507=DIRECTION ( 'NONE',  ( -0.7071067811865487940, -0.5000000000000003331, 0.4999999999999979461 ) ) ;
#13508=CARTESIAN_POINT ( 'NONE',  ( -5.800000000000006928, 29.47747564417435484, 56.65425233947093631 ) ) ;
#13517=ORIENTED_EDGE ( 'NONE', *, *, #17527, .T. ) ;
#13518=ORIENTED_EDGE ( 'NONE', *, *, #17427, .F. ) ;
#13523=ORIENTED_EDGE ( 'NONE', *, *, #13010, .T. ) ;
#13537=CARTESIAN_POINT ( 'NONE',  ( -9.120482147295685276E-15, 33.84386001800124433, 52.64142135623733054 ) ) ;
#13546=CARTESIAN_POINT ( 'NONE',  ( 4.042620306204079306, 32.68389060951040648, 53.80012125920699617 ) ) ;
#13552=CARTESIAN_POINT ( 'NONE',  ( 4.101219330881969327, 32.64264068711926825, 53.84264068711931372 ) ) ;
#13573=LINE ( 'NONE', #12002, #17199 ) ;
#13582=DIRECTION ( 'NONE',  ( 0.000000000000000000, -0.7071067811865457964, -0.7071067811865492381 ) ) ;
#13584=EDGE_LOOP ( 'NONE', ( #6847, #6057, #18738, #5819 ) ) ;
#13595=ORIENTED_EDGE ( 'NONE', *, *, #12470, .T. ) ;
#13601=AXIS2_PLACEMENT_3D ( 'NONE', #10018, #5436, #14444 ) ;
#13620=ORIENTED_EDGE ( 'NONE', *, *, #5541, .F. ) ;
#13628=LINE ( 'NONE', #1388, #4562 ) ;
#13639=ORIENTED_EDGE ( 'NONE', *, *, #5061, .T. ) ;
#13641=AXIS2_PLACEMENT_3D ( 'NONE', #2288, #13145, #3855 ) ;
#13643=DIRECTION ( 'NONE',  ( -0.000000000000000000, 0.7071067811865456854, 0.7071067811865493491 ) ) ;
#13654=AXIS2_PLACEMENT_3D ( 'NONE', #13677, #1340, #256 ) ;
#13656=CARTESIAN_POINT ( 'NONE',  ( 4.189607678530260948, 26.72836399182260791, 59.40336399182267257 ) ) ;
#13677=CARTESIAN_POINT ( 'NONE',  ( -1.040834085586084257E-14, 29.74264068711926257, 56.74264068711929809 ) ) ;
#13708=ORIENTED_EDGE ( 'NONE', *, *, #15989, .F. ) ;
#13713=CARTESIAN_POINT ( 'NONE',  ( 0.000000000000000000, 0.000000000000000000, 0.000000000000000000 ) ) ;
#13714=ORIENTED_EDGE ( 'NONE', *, *, #5814, .F. ) ;
#13724=CARTESIAN_POINT ( 'NONE',  ( -1.040834085586084257E-14, 29.74264068711926257, 56.74264068711929809 ) ) ;
#13728=LINE ( 'NONE', #591, #7157 ) ;
#13734=B_SPLINE_CURVE_WITH_KNOTS ( 'NONE', 3,
 ( #15742, #2304, #19059, #17591 ),
 .UNSPECIFIED., .F., .F.,
 ( 4, 4 ),
 ( 0.000000000000000000, 1.000000000000000000 ),
 .UNSPECIFIED. ) ;
#13748=FACE_OUTER_BOUND ( 'NONE', #13020, .T. ) ;
#13749=VERTEX_POINT ( 'NONE', #4847 ) ;
#13751=DIRECTION ( 'NONE',  ( 7.602811950582247805E-15, 0.000000000000000000, -1.000000000000000000 ) ) ;
#13782=LINE ( 'NONE', #9080, #9865 ) ;
#13784=ORIENTED_EDGE ( 'NONE', *, *, #5181, .T. ) ;
#13793=CARTESIAN_POINT ( 'NONE',  ( -3.400000000000017675, 29.83102903476760659, 56.65425233947095762 ) ) ;
#13805=DIRECTION ( 'NONE',  ( 2.775557561562891844E-16, 0.7071067811865453523, 0.7071067811865497932 ) ) ;
#13808=ORIENTED_EDGE ( 'NONE', *, *, #10931, .F. ) ;
#13809=ORIENTED_EDGE ( 'NONE', *, *, #17416, .T. ) ;
#13849=AXIS2_PLACEMENT_3D ( 'NONE', #10822, #12592, #12395 ) ;
#13854=CARTESIAN_POINT ( 'NONE',  ( -5.800000000000006928, 29.47747564417435484, 56.65425233947093631 ) ) ;
#13860=FILL_AREA_STYLE ('',( #10909 ) ) ;
#13894=DIRECTION ( 'NONE',  ( -0.7071067811865437980, 0.5000000000000043299, -0.5000000000000008882 ) ) ;
#13930=LINE ( 'NONE', #6098, #14929 ) ;
#13953=CARTESIAN_POINT ( 'NONE',  ( 4.189607678530260948, 26.72836399182260791, 59.40336399182267257 ) ) ;
#13954=ADVANCED_FACE ( 'NONE', ( #807 ), #15898, .T. ) ;
#13973=EDGE_CURVE ( 'NONE', #89, #16741, #5505, .T. ) ;
#13983=VECTOR ( 'NONE', #6689, 999.9999999999998863 ) ;
#14021=DIRECTION ( 'NONE',  ( -0.000000000000000000, 0.7071067811865456854, 0.7071067811865493491 ) ) ;
#14052=AXIS2_PLACEMENT_3D ( 'NONE', #666, #15936, #17410 ) ;
#14059=EDGE_CURVE ( 'NONE', #17432, #3008, #7069, .T. ) ;
#14079=CIRCLE ( 'NONE', #6579, 6.799999999999999822 ) ;
#14081=ADVANCED_FACE ( 'NONE', ( #19329 ), #7268, .T. ) ;
#14083=APPLICATION_CONTEXT ( 'automotive_design' ) ;
#14084=ADVANCED_FACE ( 'NONE', ( #13235 ), #2950, .T. ) ;
#14094=CARTESIAN_POINT ( 'NONE',  ( -0.1250000000000104083, 25.46464466094064250, 60.66708332270462734 ) ) ;
#14104=ORIENTED_EDGE ( 'NONE', *, *, #1714, .F. ) ;
#14108=EDGE_CURVE ( 'NONE', #5479, #6083, #8926, .T. ) ;
#14187=DIRECTION ( 'NONE',  ( 0.000000000000000000, -0.7071067811865493491, 0.7071067811865457964 ) ) ;
#14195=ORIENTED_EDGE ( 'NONE', *, *, #1360, .T. ) ;
#14216=LINE ( 'NONE', #12452, #16908 ) ;
#14218=EDGE_CURVE ( 'NONE', #1789, #3990, #4329, .T. ) ;
#14223=VERTEX_POINT ( 'NONE', #8725 ) ;
#14234=DIRECTION ( 'NONE',  ( -1.000000000000000000, 2.665111688417744333E-15, -2.272588573746785565E-15 ) ) ;
#14241=DIRECTION ( 'NONE',  ( 0.7071067811865535679, 0.4999999999999973355, -0.4999999999999940048 ) ) ;
#14257=CARTESIAN_POINT ( 'NONE',  ( 0.08838834764830767743, 29.68014068711926257, 56.80514068711929809 ) ) ;
#14262=EDGE_CURVE ( 'NONE', #4388, #5200, #13628, .T. ) ;
#14270=EDGE_CURVE ( 'NONE', #3008, #5563, #10979, .T. ) ;
#14286=VERTEX_POINT ( 'NONE', #18450 ) ;
#14325=VERTEX_POINT ( 'NONE', #18554 ) ;
#14341=CARTESIAN_POINT ( 'NONE',  ( 2.315774708385922587, 27.80336399182260720, 58.32836399182267684 ) ) ;
#14363=EDGE_LOOP ( 'NONE', ( #16681, #1357, #13311, #10645 ) ) ;
#14368=CARTESIAN_POINT ( 'NONE',  ( -4.012830983233701687, 26.60336399182265055, 59.52836399182262994 ) ) ;
#14377=VECTOR ( 'NONE', #15430, 1000.000000000000000 ) ;
#14379=VECTOR ( 'NONE', #7738, 1000.000000000000114 ) ;
#14396=LINE ( 'NONE', #3913, #4361 ) ;
#14434=EDGE_LOOP ( 'NONE', ( #9217, #14680, #468, #16320 ) ) ;
#14444=DIRECTION ( 'NONE',  ( -0.000000000000000000, 0.000000000000000000, 1.000000000000000000 ) ) ;
#14458=( NAMED_UNIT ( * ) SI_UNIT ( $, .STERADIAN. ) SOLID_ANGLE_UNIT ( ) );
#14467=CARTESIAN_POINT ( 'NONE',  ( -5.800000000000006928, 29.65425233947099315, 56.47747564417430510 ) ) ;
#14469=FACE_OUTER_BOUND ( 'NONE', #16760, .T. ) ;
#14471=CIRCLE ( 'NONE', #1965, 5.800000000000007816 ) ;
#14499=ORIENTED_EDGE ( 'NONE', *, *, #14218, .F. ) ;
#14500=ORIENTED_EDGE ( 'NONE', *, *, #9598, .F. ) ;
#14505=ORIENTED_EDGE ( 'NONE', *, *, #16594, .F. ) ;
#14511=EDGE_CURVE ( 'NONE', #6570, #1789, #267, .T. ) ;
#14532=MECHANICAL_DESIGN_GEOMETRIC_PRESENTATION_REPRESENTATION('',(#17058),#19246);
#14575=ORIENTED_EDGE ( 'NONE', *, *, #2432, .T. ) ;
#14596=ADVANCED_BREP_SHAPE_REPRESENTATION ( '', ( #10129, #1791 ), #2636 ) ;
#14632=DIRECTION ( 'NONE',  ( 0.5773502691896176264, -0.8164965809277319186, 0.000000000000000000 ) ) ;
#14634=CARTESIAN_POINT ( 'NONE',  ( -0.1250000000000104083, 32.14680374315353362, 54.33847763108504125 ) ) ;
#14639=CARTESIAN_POINT ( 'NONE',  ( -1.040834085586084257E-14, 29.74264068711925901, 56.74264068711929809 ) ) ;
#14645=CARTESIAN_POINT ( 'NONE',  ( 4.160453206537118476, 26.88344170207930617, 59.60057016663805740 ) ) ;
#14648=CARTESIAN_POINT ( 'NONE',  ( -4.012830983233701687, 26.60336399182265055, 59.52836399182262994 ) ) ;
#14658=CARTESIAN_POINT ( 'NONE',  ( -0.1250000000000104083, 31.97002704785689531, 54.16170093578840294 ) ) ;
#14659=PLANE ( 'NONE',  #4974 ) ;
#14680=ORIENTED_EDGE ( 'NONE', *, *, #2928, .F. ) ;
#14686=CARTESIAN_POINT ( 'NONE',  ( -4.189607678530337331, 26.72836399182265055, 59.40336399182262284 ) ) ;
#14692=VECTOR ( 'NONE', #3825, 1000.000000000000000 ) ;
#14711=PLANE ( 'NONE',  #3760 ) ;
#14712=ORIENTED_EDGE ( 'NONE', *, *, #6309, .T. ) ;
#14738=DIRECTION ( 'NONE',  ( -0.7071067811865561215, -0.4999999999999953926, 0.4999999999999925060 ) ) ;
#14759=AXIS2_PLACEMENT_3D ( 'NONE', #5268, #2701, #11506 ) ;
#14771=CARTESIAN_POINT ( 'NONE',  ( -1.040834085586084257E-14, 25.64142135623728080, 60.84386001800126564 ) ) ;
#14807=ORIENTED_EDGE ( 'NONE', *, *, #1003, .T. ) ;
#14820=DIRECTION ( 'NONE',  ( 0.7071067811865414665, -0.5000000000000057732, 0.5000000000000028866 ) ) ;
#14823=CARTESIAN_POINT ( 'NONE',  ( -4.101219330881938241, 32.64264068711930378, 53.84264068711927109 ) ) ;
#14879=VECTOR ( 'NONE', #2094, 1000.000000000000000 ) ;
#14906=CARTESIAN_POINT ( 'NONE',  ( 2.492551403682558675, 28.10514068711924196, 58.38014068711930804 ) ) ;
#14907=CARTESIAN_POINT ( 'NONE',  ( -0.1250000000000104083, 33.66708332270461312, 52.46464466094069934 ) ) ;
#14911=VECTOR ( 'NONE', #5375, 1000.000000000000000 ) ;
#14914=VECTOR ( 'NONE', #2883, 1000.000000000000114 ) ;
#14929=VECTOR ( 'NONE', #8065, 1000.000000000000114 ) ;
#14932=EDGE_CURVE ( 'NONE', #4327, #14325, #13782, .T. ) ;
#14982=CARTESIAN_POINT ( 'NONE',  ( -2.081668171172168513E-14, 16.06586399182267755, 70.06586399182252478 ) ) ;
#14985=PLANE ( 'NONE',  #13291 ) ;
#14987=CARTESIAN_POINT ( 'NONE',  ( 4.101219330881941794, 26.84264068711924267, 59.64264068711931088 ) ) ;
#15023=VECTOR ( 'NONE', #1175, 1000.000000000000114 ) ;
#15064=VECTOR ( 'NONE', #11668, 1000.000000000000000 ) ;
#15075=LINE ( 'NONE', #2811, #4737 ) ;
#15096=ORIENTED_EDGE ( 'NONE', *, *, #861, .F. ) ;
#15106=DIRECTION ( 'NONE',  ( 0.000000000000000000, -0.7071067811865456854, -0.7071067811865493491 ) ) ;
#15112=ORIENTED_EDGE ( 'NONE', *, *, #2657, .T. ) ;
#15127=EDGE_CURVE ( 'NONE', #19340, #2343, #8290, .T. ) ;
#15160=PLANE ( 'NONE',  #15712 ) ;
#15164=B_SPLINE_CURVE_WITH_KNOTS ( 'NONE', 3,
 ( #11896, #14645, #8570, #4363 ),
 .UNSPECIFIED., .F., .F.,
 ( 4, 4 ),
 ( 0.000000000000000000, 1.000000000000000000 ),
 .UNSPECIFIED. ) ;
#15184=VECTOR ( 'NONE', #10431, 1000.000000000000000 ) ;
#15198=VECTOR ( 'NONE', #19230, 1000.000000000000000 ) ;
#15199=ORIENTED_EDGE ( 'NONE', *, *, #17193, .F. ) ;
#15214=VECTOR ( 'NONE', #6858, 1000.000000000000000 ) ;
#15227=CARTESIAN_POINT ( 'NONE',  ( 5.800448837981379668, 29.71286850494547593, 56.77177811653250217 ) ) ;
#15232=ORIENTED_EDGE ( 'NONE', *, *, #14270, .T. ) ;
#15233=CARTESIAN_POINT ( 'NONE',  ( -9.698045712355376814E-15, 25.64142135623727370, 60.84386001800126564 ) ) ;
#15239=DIRECTION ( 'NONE',  ( 2.775557561562890858E-16, 0.7071067811865454633, 0.7071067811865496822 ) ) ;
#15244=EDGE_CURVE ( 'NONE', #13749, #5786, #9560, .T. ) ;
#15250=CARTESIAN_POINT ( 'NONE',  ( -5.800000000000006928, 29.47747564417435484, 56.65425233947093631 ) ) ;
#15264=EDGE_CURVE ( 'NONE', #9938, #16495, #2399, .T. ) ;
#15296=DIRECTION ( 'NONE',  ( -2.775557561562890858E-16, 0.7071067811865456854, 0.7071067811865493491 ) ) ;
#15314=CARTESIAN_POINT ( 'NONE',  ( -2.315774708385978098, 27.80336399182263563, 58.32836399182264131 ) ) ;
#15318=VECTOR ( 'NONE', #18002, 1000.000000000000000 ) ;
#15322=CARTESIAN_POINT ( 'NONE',  ( -2.492551403682614186, 27.92836399182264273, 58.20336399182264131 ) ) ;
#15327=EDGE_CURVE ( 'NONE', #106, #15466, #19164, .T. ) ;
#15362=EDGE_CURVE ( 'NONE', #16765, #15802, #15164, .T. ) ;
#15373=ORIENTED_EDGE ( 'NONE', *, *, #1092, .F. ) ;
#15392=AXIS2_PLACEMENT_3D ( 'NONE', #18527, #13805, #475 ) ;
#15424=ORIENTED_EDGE ( 'NONE', *, *, #13973, .T. ) ;
#15430=DIRECTION ( 'NONE',  ( -0.000000000000000000, -0.7071067811865493491, 0.7071067811865456854 ) ) ;
#15436=CARTESIAN_POINT ( 'NONE',  ( 4.189607678530287593, 32.40336399182262284, 53.72836399182268252 ) ) ;
#15466=VERTEX_POINT ( 'NONE', #2781 ) ;
#15475=VECTOR ( 'NONE', #9632, 1000.000000000000114 ) ;
#15476=CARTESIAN_POINT ( 'NONE',  ( -1.040834085586084257E-14, 29.74264068711925901, 56.74264068711929809 ) ) ;
#15491=ORIENTED_EDGE ( 'NONE', *, *, #4085, .F. ) ;
#15499=DIRECTION ( 'NONE',  ( 0.7071067811865389130, -0.5000000000000073275, 0.5000000000000048850 ) ) ;
#15505=CARTESIAN_POINT ( 'NONE',  ( -3.400000000000017675, 29.65425233947097183, 56.47747564417432642 ) ) ;
#15513=EDGE_CURVE ( 'NONE', #18191, #14223, #11596, .T. ) ;
#15532=VECTOR ( 'NONE', #8311, 1000.000000000000000 ) ;
#15546=VECTOR ( 'NONE', #15645, 1000.000000000000000 ) ;
#15549=LINE ( 'NONE', #2119, #11946 ) ;
#15567=LINE ( 'NONE', #12328, #3177 ) ;
#15575=ORIENTED_EDGE ( 'NONE', *, *, #1702, .T. ) ;
#15580=ORIENTED_EDGE ( 'NONE', *, *, #1658, .F. ) ;
#15586=ORIENTED_EDGE ( 'NONE', *, *, #4764, .T. ) ;
#15590=CARTESIAN_POINT ( 'NONE',  ( 0.1249999999999895917, 29.74264068711926257, 56.74264068711929809 ) ) ;
#15609=EDGE_LOOP ( 'NONE', ( #18621, #10305, #11350, #15424 ) ) ;
#15624=AXIS2_PLACEMENT_3D ( 'NONE', #12494, #1724, #1823 ) ;
#15645=DIRECTION ( 'NONE',  ( 1.000000000000000000, 0.000000000000000000, 0.000000000000000000 ) ) ;
#15649=SHAPE_REPRESENTATION_RELATIONSHIP ( 'NONE' , 'NONE' ,  #2502, #14596 ) ;
#15668=DIRECTION ( 'NONE',  ( -0.000000000000000000, 0.7071067811865452413, 0.7071067811865497932 ) ) ;
#15674=AXIS2_PLACEMENT_3D ( 'NONE', #4157, #11582, #14632 ) ;
#15688=PLANE ( 'NONE',  #9071 ) ;
#15703=VECTOR ( 'NONE', #4827, 1000.000000000000000 ) ;
#15712=AXIS2_PLACEMENT_3D ( 'NONE', #16731, #9270, #4234 ) ;
#15728=ORIENTED_EDGE ( 'NONE', *, *, #4571, .T. ) ;
#15742=CARTESIAN_POINT ( 'NONE',  ( 5.799326430397230503, 29.83055285973283333, 56.65377616443626607 ) ) ;
#15790=CARTESIAN_POINT ( 'NONE',  ( -0.1250000000000104083, 25.64142146683625612, 60.84290755733282197 ) ) ;
#15802=VERTEX_POINT ( 'NONE', #533 ) ;
#15811=CARTESIAN_POINT ( 'NONE',  ( -9.098294960646575315E-15, 29.83102903476757817, 56.65425233947097894 ) ) ;
#15837=( LENGTH_UNIT ( ) NAMED_UNIT ( * ) SI_UNIT ( .MILLI., .METRE. ) );
#15850=CARTESIAN_POINT ( 'NONE',  ( -1.040834085586084257E-14, 25.49999999999998934, 52.50000000000000000 ) ) ;
#15854=EDGE_CURVE ( 'NONE', #15466, #11383, #17010, .T. ) ;
#15877=FACE_OUTER_BOUND ( 'NONE', #15609, .T. ) ;
#15894=CARTESIAN_POINT ( 'NONE',  ( 5.799999999999985612, 29.65425233947092920, 56.47747564417436195 ) ) ;
#15898=PLANE ( 'NONE',  #2654 ) ;
#15902=EDGE_CURVE ( 'NONE', #12841, #6570, #1189, .T. ) ;
#15906=EDGE_LOOP ( 'NONE', ( #11057, #12950, #17340, #7528, #16962 ) ) ;
#15927=AXIS2_PLACEMENT_3D ( 'NONE', #6630, #12305, #6529 ) ;
#15936=DIRECTION ( 'NONE',  ( 3.493455720571401687E-15, 0.7071067811865496822, -0.7071067811865454633 ) ) ;
#15945=EDGE_CURVE ( 'NONE', #5878, #17254, #18883, .T. ) ;
#15954=AXIS2_PLACEMENT_3D ( 'NONE', #14368, #1232, #7212 ) ;
#15959=VECTOR ( 'NONE', #5199, 1000.000000000000000 ) ;
#15989=EDGE_CURVE ( 'NONE', #5479, #13749, #4439, .T. ) ;
#15997=VERTEX_POINT ( 'NONE', #18456 ) ;
#15999=EDGE_CURVE ( 'NONE', #8744, #576, #1339, .T. ) ;
#16035=PLANE ( 'NONE',  #1640 ) ;
#16046=VERTEX_POINT ( 'NONE', #10889 ) ;
#16062=FACE_OUTER_BOUND ( 'NONE', #4907, .T. ) ;
#16134=CARTESIAN_POINT ( 'NONE',  ( 19.09188309203663891, 29.56586399182256741, 56.56586399182270952 ) ) ;
#16139=CARTESIAN_POINT ( 'NONE',  ( 3.399999999999996803, 29.65425233947092920, 56.47747564417434774 ) ) ;
#16159=PLANE ( 'NONE',  #18131 ) ;
#16160=DIRECTION ( 'NONE',  ( -1.048036716171419796E-14, -0.7071067811865496822, 0.7071067811865454633 ) ) ;
#16183=CARTESIAN_POINT ( 'NONE',  ( 0.08838834764830674762, 29.80514068711925901, 56.68014068711929809 ) ) ;
#16187=ADVANCED_FACE ( 'NONE', ( #789 ), #18560, .T. ) ;
#16201=EDGE_CURVE ( 'NONE', #17270, #5689, #13930, .T. ) ;
#16224=CARTESIAN_POINT ( 'NONE',  ( -4.012830983233618198, 32.52836399182267257, 53.60336399182263989 ) ) ;
#16231=CARTESIAN_POINT ( 'NONE',  ( 4.012354697599942455, 32.70432772728315740, 53.78000129688596331 ) ) ;
#16253=PLANE ( 'NONE',  #9975 ) ;
#16291=UNCERTAINTY_MEASURE_WITH_UNIT (LENGTH_MEASURE( 1.000000000000000082E-05 ), #11213, 'distance_accuracy_value', 'NONE');
#16300=ORIENTED_EDGE ( 'NONE', *, *, #1702, .F. ) ;
#16309=DIRECTION ( 'NONE',  ( -0.000000000000000000, 0.000000000000000000, -1.000000000000000000 ) ) ;
#16314=VECTOR ( 'NONE', #13507, 1000.000000000000000 ) ;
#16318=CARTESIAN_POINT ( 'NONE',  ( -5.800000000000006928, 29.65425233947099315, 56.47747564417430510 ) ) ;
#16320=ORIENTED_EDGE ( 'NONE', *, *, #14262, .T. ) ;
#16328=CARTESIAN_POINT ( 'NONE',  ( 0.08332044287237951041, 33.84354269072930776, 52.64046917798810910 ) ) ;
#16340=ADVANCED_FACE ( 'NONE', ( #3448 ), #12456, .T. ) ;
#16362=LINE ( 'NONE', #9000, #14379 ) ;
#16368=VERTEX_POINT ( 'NONE', #4384 ) ;
#16391=CARTESIAN_POINT ( 'NONE',  ( -4.012354697599992193, 26.78000129688593134, 59.70432772728315740 ) ) ;
#16402=ORIENTED_EDGE ( 'NONE', *, *, #16802, .T. ) ;
#16433=ADVANCED_FACE ( 'NONE', ( #8877 ), #2696, .T. ) ;
#16446=AXIS2_PLACEMENT_3D ( 'NONE', #17860, #4732, #4530 ) ;
#16470=ORIENTED_EDGE ( 'NONE', *, *, #18839, .F. ) ;
#16482=DIRECTION ( 'NONE',  ( -1.000000000000000000, 0.000000000000000000, -0.000000000000000000 ) ) ;
#16484=ORIENTED_EDGE ( 'NONE', *, *, #8356, .T. ) ;
#16495=VERTEX_POINT ( 'NONE', #6535 ) ;
#16549=VECTOR ( 'NONE', #11592, 1000.000000000000000 ) ;
#16565=AXIS2_PLACEMENT_3D ( 'NONE', #8199, #5728, #4460 ) ;
#16577=ORIENTED_EDGE ( 'NONE', *, *, #11078, .F. ) ;
#16578=CARTESIAN_POINT ( 'NONE',  ( -0.1250000000000104083, 33.66708332270461312, 52.46464466094069934 ) ) ;
#16594=EDGE_CURVE ( 'NONE', #15997, #17726, #4061, .T. ) ;
#16597=VECTOR ( 'NONE', #9169, 999.9999999999998863 ) ;
#16598=CARTESIAN_POINT ( 'NONE',  ( -1.040834085586084257E-14, 25.64142135623728080, 60.84386001800126564 ) ) ;
#16599=EDGE_CURVE ( 'NONE', #5689, #2281, #13734, .T. ) ;
#16627=DIRECTION ( 'NONE',  ( 0.000000000000000000, -0.7071067811865495711, 0.7071067811865454633 ) ) ;
#16645=VECTOR ( 'NONE', #3798, 1000.000000000000114 ) ;
#16657=CARTESIAN_POINT ( 'NONE',  ( 4.189607678530260948, 26.72836399182260791, 59.40336399182267257 ) ) ;
#16663=DIRECTION ( 'NONE',  ( -0.7071067811865437980, 0.5000000000000039968, -0.5000000000000013323 ) ) ;
#16672=ORIENTED_EDGE ( 'NONE', *, *, #18284, .F. ) ;
#16681=ORIENTED_EDGE ( 'NONE', *, *, #1195, .T. ) ;
#16687=CARTESIAN_POINT ( 'NONE',  ( -0.1250000000000104083, 33.84290755733280776, 52.64142146683631296 ) ) ;
#16699=LINE ( 'NONE', #3265, #3514 ) ;
#16731=CARTESIAN_POINT ( 'NONE',  ( 2.315774708385922587, 27.80336399182260720, 58.32836399182267684 ) ) ;
#16741=VERTEX_POINT ( 'NONE', #5733 ) ;
#16755=LINE ( 'NONE', #1559, #17500 ) ;
#16759=CARTESIAN_POINT ( 'NONE',  ( -4.012830983233618198, 32.52836399182267257, 53.60336399182263989 ) ) ;
#16760=EDGE_LOOP ( 'NONE', ( #5039, #6412, #3129, #11730 ) ) ;
#16762=VERTEX_POINT ( 'NONE', #11794 ) ;
#16765=VERTEX_POINT ( 'NONE', #17786 ) ;
#16802=EDGE_CURVE ( 'NONE', #7943, #4327, #10516, .T. ) ;
#16824=FACE_OUTER_BOUND ( 'NONE', #11053, .T. ) ;
#16855=DIRECTION ( 'NONE',  ( 0.000000000000000000, -0.7071067811865493491, 0.7071067811865457964 ) ) ;
#16864=ORIENTED_EDGE ( 'NONE', *, *, #5052, .T. ) ;
#16908=VECTOR ( 'NONE', #14021, 1000.000000000000000 ) ;
#16911=EDGE_CURVE ( 'NONE', #16046, #3132, #4953, .T. ) ;
#16923=AXIS2_PLACEMENT_3D ( 'NONE', #13724, #5015, #3631 ) ;
#16929=VECTOR ( 'NONE', #6312, 1000.000000000000000 ) ;
#16934=VERTEX_POINT ( 'NONE', #2188 ) ;
#16960=ADVANCED_FACE ( 'NONE', ( #7989 ), #6614, .T. ) ;
#16962=ORIENTED_EDGE ( 'NONE', *, *, #15945, .F. ) ;
#17010=LINE ( 'NONE', #15811, #19306 ) ;
#17030=DIRECTION ( 'NONE',  ( -0.000000000000000000, 0.7071067811865456854, 0.7071067811865493491 ) ) ;
#17058=STYLED_ITEM ( 'NONE', ( #11403 ), #14596 ) ;
#17102=VECTOR ( 'NONE', #742, 1000.000000000000000 ) ;
#17121=CARTESIAN_POINT ( 'NONE',  ( 5.799999999999985612, 29.47747564417429444, 56.65425233947099315 ) ) ;
#17126=CARTESIAN_POINT ( 'NONE',  ( 3.399999999999996803, 29.65425233947093631, 56.83102903476762435 ) ) ;
#17141=ORIENTED_EDGE ( 'NONE', *, *, #15327, .T. ) ;
#17160=DIRECTION ( 'NONE',  ( -0.5773502691896311712, -0.8164965809277222597, 0.000000000000000000 ) ) ;
#17178=CARTESIAN_POINT ( 'NONE',  ( 2.492551403682577771, 31.20336399182262710, 54.92836399182266405 ) ) ;
#17182=ORIENTED_EDGE ( 'NONE', *, *, #10181, .T. ) ;
#17193=EDGE_CURVE ( 'NONE', #5763, #5764, #13142, .T. ) ;
#17199=VECTOR ( 'NONE', #4575, 1000.000000000000114 ) ;
#17226=ORIENTED_EDGE ( 'NONE', *, *, #14218, .T. ) ;
#17234=DIRECTION ( 'NONE',  ( 2.220446049250313081E-16, 0.7071067811865452413, 0.7071067811865497932 ) ) ;
#17254=VERTEX_POINT ( 'NONE', #17764 ) ;
#17257=LINE ( 'NONE', #3635, #14692 ) ;
#17270=VERTEX_POINT ( 'NONE', #18164 ) ;
#17273=DIRECTION ( 'NONE',  ( 0.000000000000000000, 0.7071067811865456854, 0.7071067811865494601 ) ) ;
#17311=FILL_AREA_STYLE_COLOUR ( '', #12029 ) ;
#17325=CARTESIAN_POINT ( 'NONE',  ( 0.1249999999999895917, 27.16170093578836031, 58.97002704785691662 ) ) ;
#17331=EDGE_LOOP ( 'NONE', ( #4805, #286, #7120, #17773 ) ) ;
#17340=ORIENTED_EDGE ( 'NONE', *, *, #861, .T. ) ;
#17350=CARTESIAN_POINT ( 'NONE',  ( 0.1249999999999895917, 27.33847763108499507, 59.14680374315354783 ) ) ;
#17360=ORIENTED_EDGE ( 'NONE', *, *, #12281, .F. ) ;
#17362=ORIENTED_EDGE ( 'NONE', *, *, #327, .F. ) ;
#17363=DIRECTION ( 'NONE',  ( -0.7071067811865414665, 0.5000000000000057732, -0.5000000000000028866 ) ) ;
#17395=DIRECTION ( 'NONE',  ( 0.000000000000000000, -7.382983113757290994E-15, -1.000000000000000000 ) ) ;
#17405=VECTOR ( 'NONE', #15668, 1000.000000000000000 ) ;
#17406=VECTOR ( 'NONE', #17030, 1000.000000000000000 ) ;
#17410=DIRECTION ( 'NONE',  ( 0.000000000000000000, 0.7071067811865454633, 0.7071067811865496822 ) ) ;
#17416=EDGE_CURVE ( 'NONE', #9861, #6083, #4618, .T. ) ;
#17424=ORIENTED_EDGE ( 'NONE', *, *, #1812, .F. ) ;
#17427=EDGE_CURVE ( 'NONE', #5563, #11653, #18829, .T. ) ;
#17429=LINE ( 'NONE', #8600, #13186 ) ;
#17432=VERTEX_POINT ( 'NONE', #5489 ) ;
#17434=VERTEX_POINT ( 'NONE', #17350 ) ;
#17446=ORIENTED_EDGE ( 'NONE', *, *, #314, .T. ) ;
#17451=CARTESIAN_POINT ( 'NONE',  ( -5.800000000000005151, 29.74264068711930520, 56.74264068711926257 ) ) ;
#17455=VERTEX_POINT ( 'NONE', #12741 ) ;
#17481=CARTESIAN_POINT ( 'NONE',  ( -5.800448907431086099, 29.80092238452525066, 56.68308948419213777 ) ) ;
#17500=VECTOR ( 'NONE', #4406, 1000.000000000000000 ) ;
#17523=ORIENTED_EDGE ( 'NONE', *, *, #545, .F. ) ;
#17527=EDGE_CURVE ( 'NONE', #5763, #14286, #11262, .T. ) ;
#17532=DIRECTION ( 'NONE',  ( -0.7071067811865437980, 0.5000000000000043299, -0.5000000000000008882 ) ) ;
#17533=CARTESIAN_POINT ( 'NONE',  ( 4.012830983233651061, 32.52836399182262994, 53.60336399182268252 ) ) ;
#17543=ORIENTED_EDGE ( 'NONE', *, *, #10599, .F. ) ;
#17546=VECTOR ( 'NONE', #6119, 1000.000000000000000 ) ;
#17557=PLANE ( 'NONE',  #609 ) ;
#17591=CARTESIAN_POINT ( 'NONE',  ( 5.799999999999984723, 29.74264068711924835, 56.74264068711931230 ) ) ;
#17624=EDGE_CURVE ( 'NONE', #11781, #1447, #4311, .T. ) ;
#17628=EDGE_LOOP ( 'NONE', ( #8945, #13518, #17543, #12805 ) ) ;
#17632=DIRECTION ( 'NONE',  ( 0.7071067811865463515, -0.5000000000000023315, 0.4999999999999994449 ) ) ;
#17674=VECTOR ( 'NONE', #12772, 1000.000000000000000 ) ;
#17691=DIRECTION ( 'NONE',  ( 0.7071067811865537900, 0.4999999999999972800, -0.4999999999999940603 ) ) ;
#17717=PRODUCT ( 'Browning Control Rotary Dial', 'Browning Control Rotary Dial', '', ( #17761 ) ) ;
#17724=CARTESIAN_POINT ( 'NONE',  ( 4.189607678530287593, 32.40336399182262284, 53.72836399182268252 ) ) ;
#17726=VERTEX_POINT ( 'NONE', #2930 ) ;
#17755=ORIENTED_EDGE ( 'NONE', *, *, #6960, .F. ) ;
#17761=PRODUCT_CONTEXT ( 'NONE', #4057, 'mechanical' ) ;
#17764=CARTESIAN_POINT ( 'NONE',  ( -4.101219330882018177, 26.84264068711928530, 59.64264068711926825 ) ) ;
#17767=ORIENTED_EDGE ( 'NONE', *, *, #10420, .T. ) ;
#17773=ORIENTED_EDGE ( 'NONE', *, *, #13213, .F. ) ;
#17774=DIRECTION ( 'NONE',  ( -1.048036716171419796E-14, -0.7071067811865496822, 0.7071067811865454633 ) ) ;
#17786=CARTESIAN_POINT ( 'NONE',  ( 4.189131392896553230, 26.90500129688588871, 59.57932772728319293 ) ) ;
#17797=CARTESIAN_POINT ( 'NONE',  ( 0.04165538583019195301, 33.84386001800125143, 52.64078660347674798 ) ) ;
#17802=LINE ( 'NONE', #16224, #13178 ) ;
#17814=DIRECTION ( 'NONE',  ( -1.000000000000000000, 2.470246229790980797E-15, -2.470246229790967386E-15 ) ) ;
#17835=VECTOR ( 'NONE', #17363, 1000.000000000000000 ) ;
#17843=ORIENTED_EDGE ( 'NONE', *, *, #11472, .T. ) ;
#17852=EDGE_LOOP ( 'NONE', ( #17767, #8246, #13708, #13620 ) ) ;
#17860=CARTESIAN_POINT ( 'NONE',  ( -19.09188309203666023, 29.56586399182277347, 56.56586399182251057 ) ) ;
#17863=LINE ( 'NONE', #9322, #10972 ) ;
#17868=AXIS2_PLACEMENT_3D ( 'NONE', #13306, #5874, #11945 ) ;
#17882=EDGE_CURVE ( 'NONE', #16762, #4322, #9105, .T. ) ;
#17916=ORIENTED_EDGE ( 'NONE', *, *, #18600, .T. ) ;
#17919=EDGE_CURVE ( 'NONE', #17455, #885, #18897, .T. ) ;
#17931=CARTESIAN_POINT ( 'NONE',  ( -1.040834085586084257E-14, 29.74264068711925901, 56.74264068711929809 ) ) ;
#17958=DIRECTION ( 'NONE',  ( -0.7071067811865463515, 0.5000000000000024425, -0.4999999999999993339 ) ) ;
#17959=DIRECTION ( 'NONE',  ( 2.775557561562890858E-16, 0.7071067811865454633, 0.7071067811865496822 ) ) ;
#17960=B_SPLINE_CURVE_WITH_KNOTS ( 'NONE', 3,
 ( #7578, #13546, #3165, #125 ),
 .UNSPECIFIED., .F., .F.,
 ( 4, 4 ),
 ( 0.000000000000000000, 1.000000000000000000 ),
 .UNSPECIFIED. ) ;
#17977=CARTESIAN_POINT ( 'NONE',  ( -4.189607678530257395, 32.40336399182267257, 53.72836399182263278 ) ) ;
#17978=LINE ( 'NONE', #336, #17546 ) ;
#17986=EDGE_CURVE ( 'NONE', #11055, #5967, #12713, .T. ) ;
#17994=EDGE_CURVE ( 'NONE', #5786, #17434, #852, .T. ) ;
#18002=DIRECTION ( 'NONE',  ( -1.000000000000000000, 0.000000000000000000, 0.000000000000000000 ) ) ;
#18010=PLANE ( 'NONE',  #18979 ) ;
#18026=ORIENTED_EDGE ( 'NONE', *, *, #14270, .F. ) ;
#18036=AXIS2_PLACEMENT_3D ( 'NONE', #8782, #11921, #11194 ) ;
#18109=ORIENTED_EDGE ( 'NONE', *, *, #17919, .T. ) ;
#18131=AXIS2_PLACEMENT_3D ( 'NONE', #2730, #2825, #1263 ) ;
#18159=VECTOR ( 'NONE', #3699, 1000.000000000000114 ) ;
#18164=CARTESIAN_POINT ( 'NONE',  ( 5.799999999999985612, 29.65425233947092920, 56.47747564417436195 ) ) ;
#18183=AXIS2_PLACEMENT_3D ( 'NONE', #12981, #2503, #14187 ) ;
#18184=PLANE ( 'NONE',  #7833 ) ;
#18191=VERTEX_POINT ( 'NONE', #16139 ) ;
#18215=ORIENTED_EDGE ( 'NONE', *, *, #15902, .F. ) ;
#18242=EDGE_LOOP ( 'NONE', ( #305, #3212, #15232, #8502 ) ) ;
#18261=CARTESIAN_POINT ( 'NONE',  ( 0.1249999999999895917, 31.97002704785689531, 54.16170093578840294 ) ) ;
#18269=ADVANCED_FACE ( 'NONE', ( #13383 ), #5950, .T. ) ;
#18284=EDGE_CURVE ( 'NONE', #9708, #17726, #8037, .T. ) ;
#18311=ORIENTED_EDGE ( 'NONE', *, *, #6285, .T. ) ;
#18325=DIRECTION ( 'NONE',  ( -0.7071067811865486830, -0.5000000000000005551, 0.4999999999999978351 ) ) ;
#18333=ORIENTED_EDGE ( 'NONE', *, *, #5814, .T. ) ;
#18335=ORIENTED_EDGE ( 'NONE', *, *, #6336, .F. ) ;
#18350=ORIENTED_EDGE ( 'NONE', *, *, #9639, .T. ) ;
#18352=CARTESIAN_POINT ( 'NONE',  ( -0.1250000000000104083, 29.74264068711926257, 56.74264068711929809 ) ) ;
#18353=DIRECTION ( 'NONE',  ( 0.000000000000000000, 0.7071067811865456854, 0.7071067811865494601 ) ) ;
#18369=ORIENTED_EDGE ( 'NONE', *, *, #545, .T. ) ;
#18373=VECTOR ( 'NONE', #15239, 1000.000000000000114 ) ;
#18376=ORIENTED_EDGE ( 'NONE', *, *, #14932, .F. ) ;
#18383=EDGE_CURVE ( 'NONE', #1809, #5878, #1539, .T. ) ;
#18395=PLANE ( 'NONE',  #13849 ) ;
#18408=VERTEX_POINT ( 'NONE', #6051 ) ;
#18414=ADVANCED_FACE ( 'NONE', ( #9082 ), #18010, .T. ) ;
#18426=CARTESIAN_POINT ( 'NONE',  ( -4.012830983233701687, 26.60336399182265055, 59.52836399182262994 ) ) ;
#18427=FACE_OUTER_BOUND ( 'NONE', #13584, .T. ) ;
#18450=CARTESIAN_POINT ( 'NONE',  ( 2.492551403682577771, 31.38014068711926541, 55.10514068711930236 ) ) ;
#18453=CARTESIAN_POINT ( 'NONE',  ( 13.49999999999992362, 39.11180553784094371, 47.01992244580438296 ) ) ;
#18456=CARTESIAN_POINT ( 'NONE',  ( -9.120482147295685276E-15, 33.84386001800124433, 52.64142135623733054 ) ) ;
#18467=LINE ( 'NONE', #5229, #16929 ) ;
#18479=ADVANCED_FACE ( 'NONE', ( #18758 ), #11292, .T. ) ;
#18488=ADVANCED_FACE ( 'NONE', ( #10005 ), #12949, .T. ) ;
#18506=ORIENTED_EDGE ( 'NONE', *, *, #9790, .F. ) ;
#18518=FACE_OUTER_BOUND ( 'NONE', #14434, .T. ) ;
#18527=CARTESIAN_POINT ( 'NONE',  ( 13.49999999999981348, 20.01992244580421598, 66.11180553784100766 ) ) ;
#18544=CARTESIAN_POINT ( 'NONE',  ( 0.1249999999999895917, 31.97002704785689531, 54.16170093578840294 ) ) ;
#18554=CARTESIAN_POINT ( 'NONE',  ( 2.315774708385922587, 27.98014068711924551, 58.50514068711930804 ) ) ;
#18560=PLANE ( 'NONE',  #3964 ) ;
#18576=DIRECTION ( 'NONE',  ( 0.000000000000000000, -0.7071067811865493491, 0.7071067811865456854 ) ) ;
#18600=EDGE_CURVE ( 'NONE', #11781, #11383, #5425, .T. ) ;
#18621=ORIENTED_EDGE ( 'NONE', *, *, #8922, .T. ) ;
#18626=ORIENTED_EDGE ( 'NONE', *, *, #3003, .T. ) ;
#18651=AXIS2_PLACEMENT_3D ( 'NONE', #11857, #17958, #10392 ) ;
#18677=ORIENTED_EDGE ( 'NONE', *, *, #2549, .F. ) ;
#18684=LINE ( 'NONE', #10825, #17674 ) ;
#18689=VECTOR ( 'NONE', #12948, 1000.000000000000114 ) ;
#18719=FACE_OUTER_BOUND ( 'NONE', #389, .T. ) ;
#18721=CARTESIAN_POINT ( 'NONE',  ( 4.189131392896579875, 32.57932772728315740, 53.90500129688597042 ) ) ;
#18728=EDGE_LOOP ( 'NONE', ( #212, #1170, #11464, #18109 ) ) ;
#18738=ORIENTED_EDGE ( 'NONE', *, *, #5181, .F. ) ;
#18758=FACE_OUTER_BOUND ( 'NONE', #9233, .T. ) ;
#18765=CARTESIAN_POINT ( 'NONE',  ( 3.399999999999996803, 29.47747564417430155, 56.65425233947098604 ) ) ;
#18829=LINE ( 'NONE', #705, #15214 ) ;
#18839=EDGE_CURVE ( 'NONE', #14325, #5967, #10893, .T. ) ;
#18842=EDGE_LOOP ( 'NONE', ( #6849, #13219, #3343, #8918 ) ) ;
#18860=DIRECTION ( 'NONE',  ( 3.493455720571401687E-15, 0.7071067811865496822, -0.7071067811865454633 ) ) ;
#18883=B_SPLINE_CURVE_WITH_KNOTS ( 'NONE', 3,
 ( #16391, #4738, #11968, #9135 ),
 .UNSPECIFIED., .F., .F.,
 ( 4, 4 ),
 ( 0.000000000000000000, 1.000000000000000000 ),
 .UNSPECIFIED. ) ;
#18891=VERTEX_POINT ( 'NONE', #15314 ) ;
#18897=LINE ( 'NONE', #6659, #14911 ) ;
#18916=FACE_OUTER_BOUND ( 'NONE', #10671, .T. ) ;
#18979=AXIS2_PLACEMENT_3D ( 'NONE', #2191, #7716, #8185 ) ;
#18983=DIRECTION ( 'NONE',  ( 1.000000000000000000, -7.160938508832259686E-15, 7.660538869913580129E-15 ) ) ;
#18986=FACE_OUTER_BOUND ( 'NONE', #19200, .T. ) ;
#19042=PRODUCT_DEFINITION_CONTEXT ( 'detailed design', #14083, 'design' ) ;
#19050=LINE ( 'NONE', #2295, #10942 ) ;
#19059=CARTESIAN_POINT ( 'NONE',  ( 5.800448837981379668, 29.77177811653243822, 56.71286850494553988 ) ) ;
#19076=AXIS2_PLACEMENT_3D ( 'NONE', #14686, #10071, #3914 ) ;
#19105=CARTESIAN_POINT ( 'NONE',  ( -4.189607678530257395, 32.40336399182267257, 53.72836399182263278 ) ) ;
#19108=VECTOR ( 'NONE', #16663, 1000.000000000000000 ) ;
#19120=VECTOR ( 'NONE', #8925, 1000.000000000000114 ) ;
#19129=AXIS2_PLACEMENT_3D ( 'NONE', #7453, #4525, #7555 ) ;
#19164=LINE ( 'NONE', #16318, #14914 ) ;
#19200=EDGE_LOOP ( 'NONE', ( #13714, #1349 ) ) ;
#19230=DIRECTION ( 'NONE',  ( -0.000000000000000000, 0.7071067811865452413, 0.7071067811865497932 ) ) ;
#19246=( GEOMETRIC_REPRESENTATION_CONTEXT ( 3 ) GLOBAL_UNCERTAINTY_ASSIGNED_CONTEXT ( ( #7673 ) ) GLOBAL_UNIT_ASSIGNED_CONTEXT ( ( #15837, #12885, #14458 ) ) REPRESENTATION_CONTEXT ( 'NONE', 'WORKASPACE' ) );
#19252=CARTESIAN_POINT ( 'NONE',  ( 4.130991513055743525, 32.62172003681456545, 53.86292658466342687 ) ) ;
#19303=CARTESIAN_POINT ( 'NONE',  ( -2.492551403682614186, 27.92836399182264273, 58.20336399182264131 ) ) ;
#19306=VECTOR ( 'NONE', #903, 1000.000000000000000 ) ;
#19329=FACE_OUTER_BOUND ( 'NONE', #3422, .T. ) ;
#19340=VERTEX_POINT ( 'NONE', #3131 ) ;
ENDSEC;
END-ISO-10303-21;
